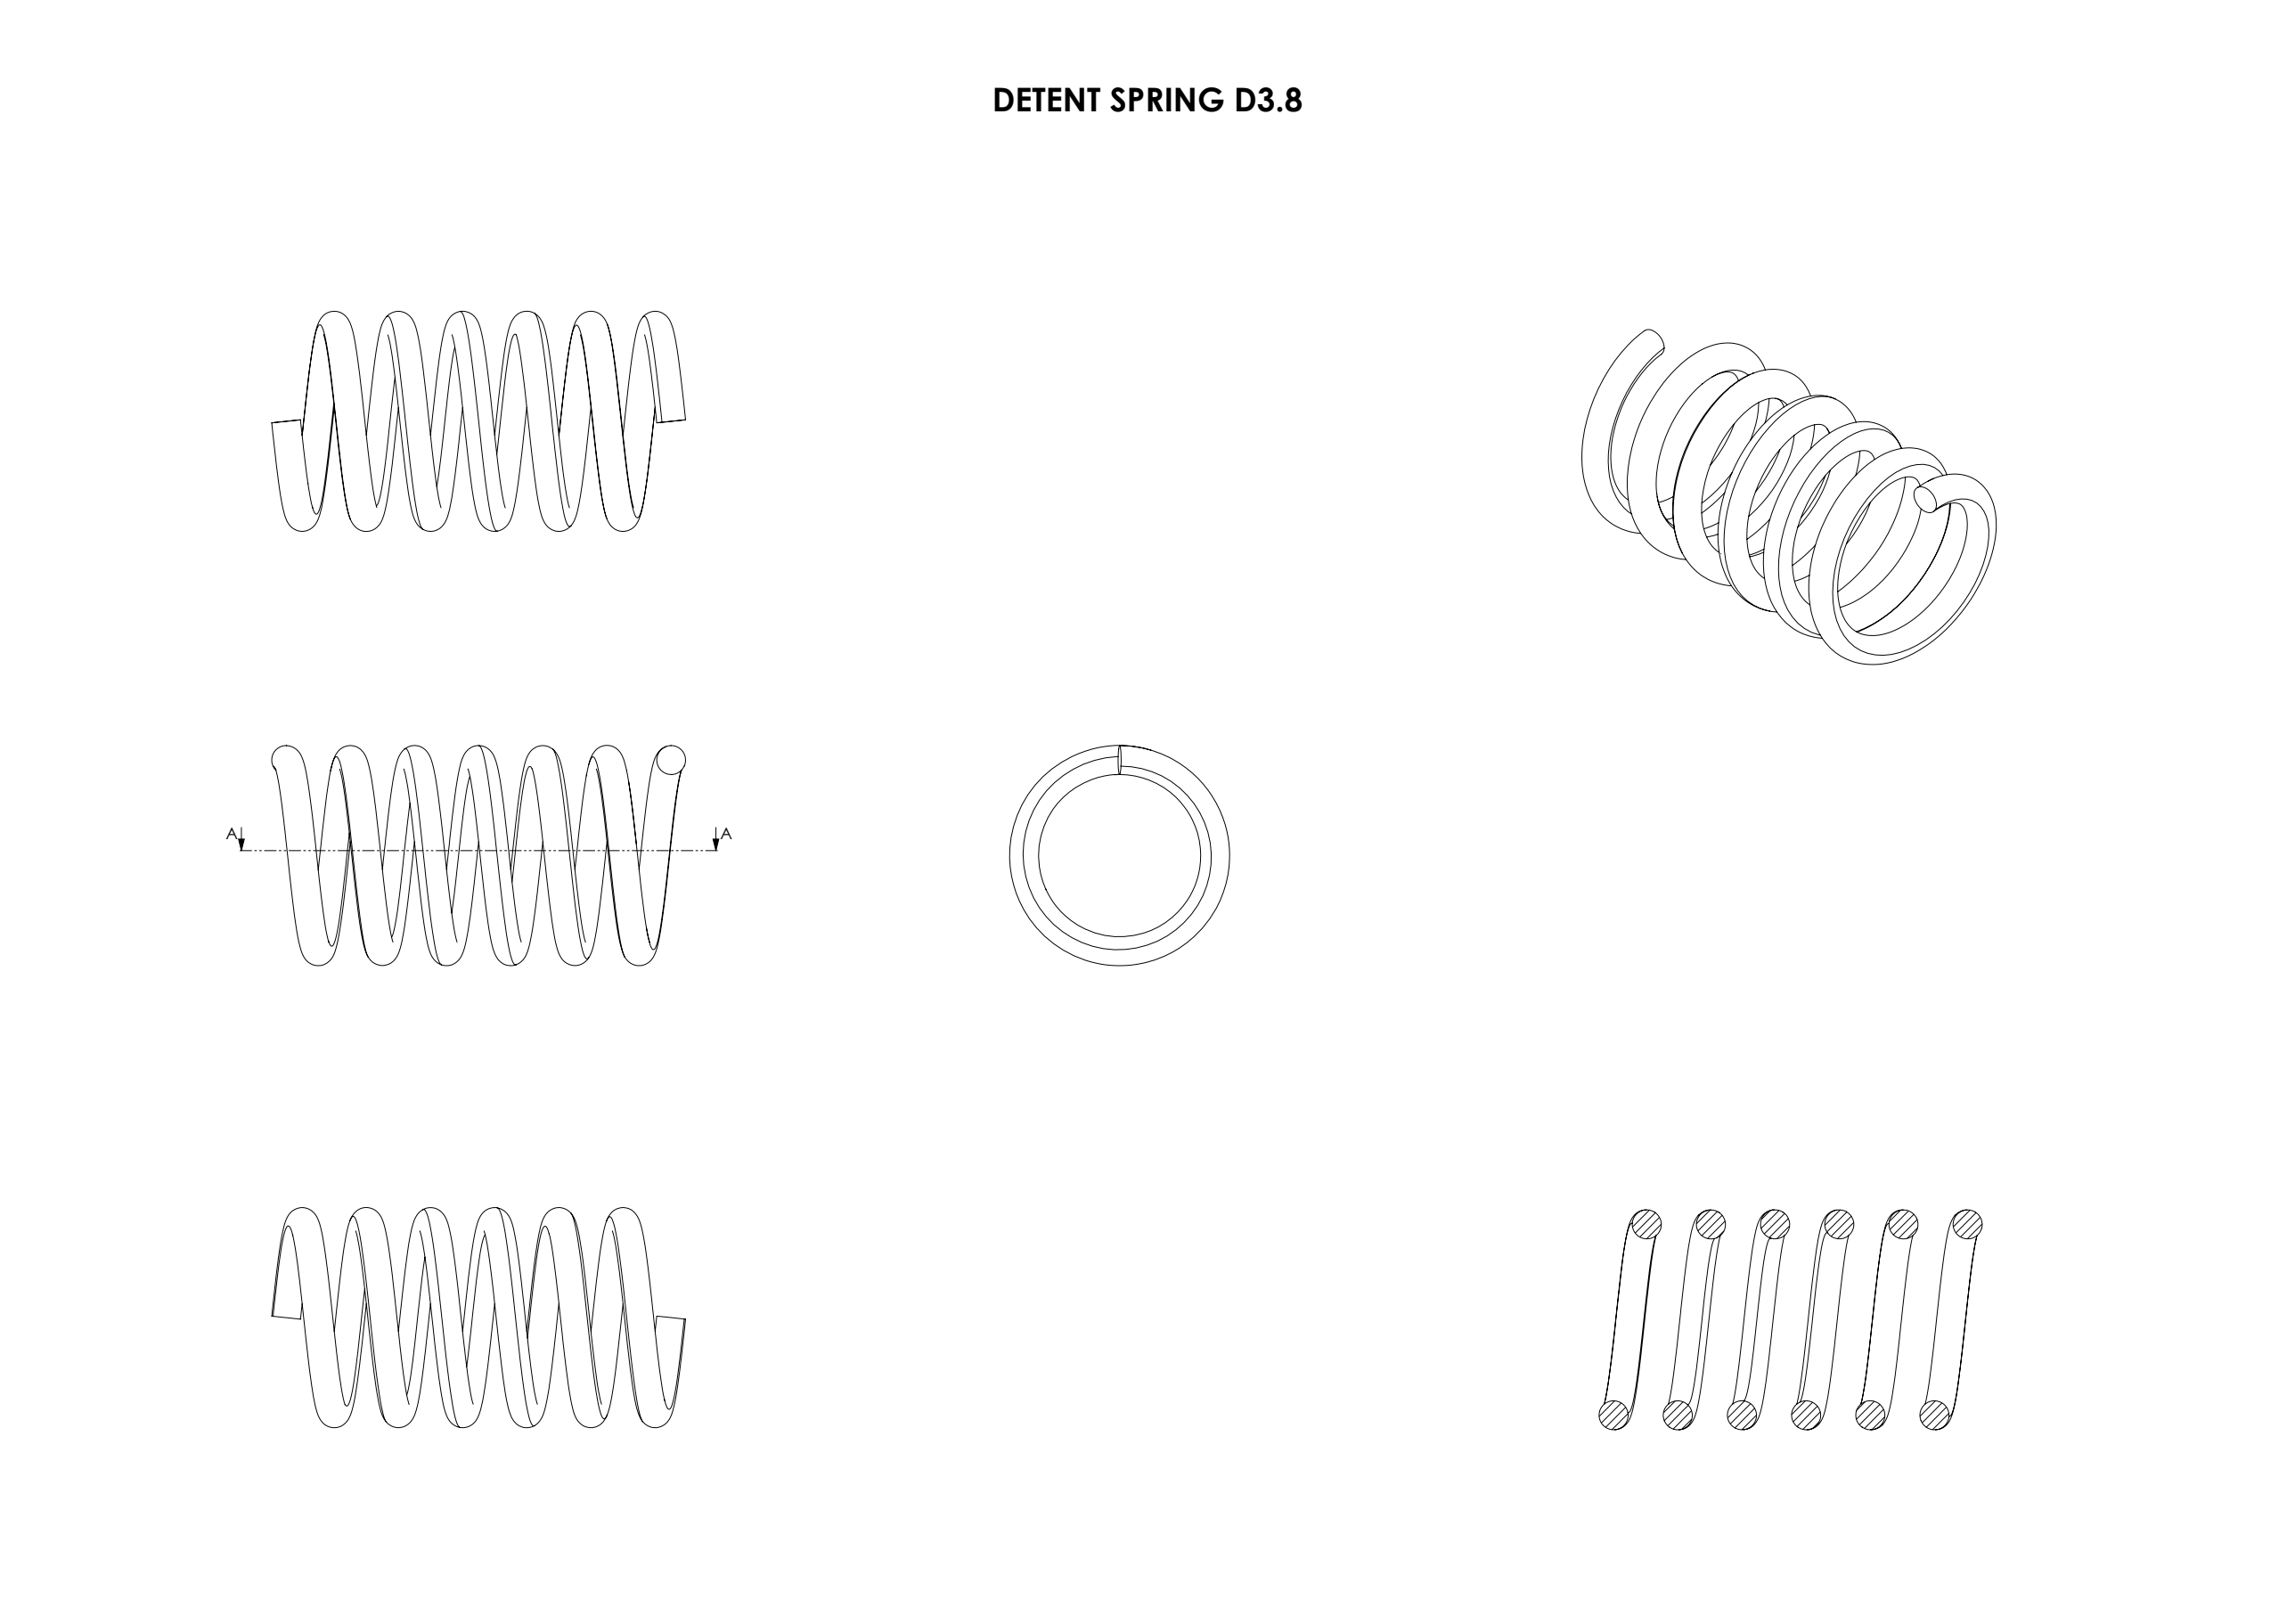
ISO-10303-21;
HEADER;
/* Generated by software containing ST-Developer
 * from STEP Tools, Inc. (www.steptools.com) 
 */

FILE_DESCRIPTION(
/* description */ (''),
/* implementation_level */ '2;1');

FILE_NAME(
/* name */ '10_Detent_Spring_D3.8.step',
/* time_stamp */ '2026-10-21T02:03:06-07:00',
/* author */ (''),
/* organization */ (''),
/* preprocessor_version */ 'ST-DEVELOPER v20.2',
/* originating_system */ 'Autodesk Translation Framework v15.15.0.0',
/* authorisation */ '');

FILE_SCHEMA (('AUTOMOTIVE_DESIGN { 1 0 10303 214 3 1 1 }'));
ENDSEC;

DATA;
#10=MECHANICAL_DESIGN_GEOMETRIC_PRESENTATION_REPRESENTATION('',(#124),#38528);
#86=B_SPLINE_SURFACE_WITH_KNOTS('',3,3,((#33827,#33828,#33829,#33830,#33831,
#33832,#33833,#33834,#33835,#33836,#33837,#33838,#33839,#33840,#33841,#33842,
#33843,#33844,#33845,#33846,#33847,#33848,#33849,#33850,#33851,#33852,#33853,
#33854,#33855,#33856,#33857,#33858,#33859,#33860,#33861,#33862,#33863,#33864,
#33865,#33866,#33867,#33868,#33869,#33870,#33871,#33872,#33873,#33874,#33875,
#33876,#33877,#33878,#33879,#33880,#33881,#33882,#33883,#33884,#33885,#33886,
#33887,#33888,#33889),(#33890,#33891,#33892,#33893,#33894,#33895,#33896,
#33897,#33898,#33899,#33900,#33901,#33902,#33903,#33904,#33905,#33906,#33907,
#33908,#33909,#33910,#33911,#33912,#33913,#33914,#33915,#33916,#33917,#33918,
#33919,#33920,#33921,#33922,#33923,#33924,#33925,#33926,#33927,#33928,#33929,
#33930,#33931,#33932,#33933,#33934,#33935,#33936,#33937,#33938,#33939,#33940,
#33941,#33942,#33943,#33944,#33945,#33946,#33947,#33948,#33949,#33950,#33951,
#33952),(#33953,#33954,#33955,#33956,#33957,#33958,#33959,#33960,#33961,
#33962,#33963,#33964,#33965,#33966,#33967,#33968,#33969,#33970,#33971,#33972,
#33973,#33974,#33975,#33976,#33977,#33978,#33979,#33980,#33981,#33982,#33983,
#33984,#33985,#33986,#33987,#33988,#33989,#33990,#33991,#33992,#33993,#33994,
#33995,#33996,#33997,#33998,#33999,#34000,#34001,#34002,#34003,#34004,#34005,
#34006,#34007,#34008,#34009,#34010,#34011,#34012,#34013,#34014,#34015),
(#34016,#34017,#34018,#34019,#34020,#34021,#34022,#34023,#34024,#34025,
#34026,#34027,#34028,#34029,#34030,#34031,#34032,#34033,#34034,#34035,#34036,
#34037,#34038,#34039,#34040,#34041,#34042,#34043,#34044,#34045,#34046,#34047,
#34048,#34049,#34050,#34051,#34052,#34053,#34054,#34055,#34056,#34057,#34058,
#34059,#34060,#34061,#34062,#34063,#34064,#34065,#34066,#34067,#34068,#34069,
#34070,#34071,#34072,#34073,#34074,#34075,#34076,#34077,#34078),(#34079,
#34080,#34081,#34082,#34083,#34084,#34085,#34086,#34087,#34088,#34089,#34090,
#34091,#34092,#34093,#34094,#34095,#34096,#34097,#34098,#34099,#34100,#34101,
#34102,#34103,#34104,#34105,#34106,#34107,#34108,#34109,#34110,#34111,#34112,
#34113,#34114,#34115,#34116,#34117,#34118,#34119,#34120,#34121,#34122,#34123,
#34124,#34125,#34126,#34127,#34128,#34129,#34130,#34131,#34132,#34133,#34134,
#34135,#34136,#34137,#34138,#34139,#34140,#34141),(#34142,#34143,#34144,
#34145,#34146,#34147,#34148,#34149,#34150,#34151,#34152,#34153,#34154,#34155,
#34156,#34157,#34158,#34159,#34160,#34161,#34162,#34163,#34164,#34165,#34166,
#34167,#34168,#34169,#34170,#34171,#34172,#34173,#34174,#34175,#34176,#34177,
#34178,#34179,#34180,#34181,#34182,#34183,#34184,#34185,#34186,#34187,#34188,
#34189,#34190,#34191,#34192,#34193,#34194,#34195,#34196,#34197,#34198,#34199,
#34200,#34201,#34202,#34203,#34204),(#34205,#34206,#34207,#34208,#34209,
#34210,#34211,#34212,#34213,#34214,#34215,#34216,#34217,#34218,#34219,#34220,
#34221,#34222,#34223,#34224,#34225,#34226,#34227,#34228,#34229,#34230,#34231,
#34232,#34233,#34234,#34235,#34236,#34237,#34238,#34239,#34240,#34241,#34242,
#34243,#34244,#34245,#34246,#34247,#34248,#34249,#34250,#34251,#34252,#34253,
#34254,#34255,#34256,#34257,#34258,#34259,#34260,#34261,#34262,#34263,#34264,
#34265,#34266,#34267),(#34268,#34269,#34270,#34271,#34272,#34273,#34274,
#34275,#34276,#34277,#34278,#34279,#34280,#34281,#34282,#34283,#34284,#34285,
#34286,#34287,#34288,#34289,#34290,#34291,#34292,#34293,#34294,#34295,#34296,
#34297,#34298,#34299,#34300,#34301,#34302,#34303,#34304,#34305,#34306,#34307,
#34308,#34309,#34310,#34311,#34312,#34313,#34314,#34315,#34316,#34317,#34318,
#34319,#34320,#34321,#34322,#34323,#34324,#34325,#34326,#34327,#34328,#34329,
#34330),(#34331,#34332,#34333,#34334,#34335,#34336,#34337,#34338,#34339,
#34340,#34341,#34342,#34343,#34344,#34345,#34346,#34347,#34348,#34349,#34350,
#34351,#34352,#34353,#34354,#34355,#34356,#34357,#34358,#34359,#34360,#34361,
#34362,#34363,#34364,#34365,#34366,#34367,#34368,#34369,#34370,#34371,#34372,
#34373,#34374,#34375,#34376,#34377,#34378,#34379,#34380,#34381,#34382,#34383,
#34384,#34385,#34386,#34387,#34388,#34389,#34390,#34391,#34392,#34393),
(#34394,#34395,#34396,#34397,#34398,#34399,#34400,#34401,#34402,#34403,
#34404,#34405,#34406,#34407,#34408,#34409,#34410,#34411,#34412,#34413,#34414,
#34415,#34416,#34417,#34418,#34419,#34420,#34421,#34422,#34423,#34424,#34425,
#34426,#34427,#34428,#34429,#34430,#34431,#34432,#34433,#34434,#34435,#34436,
#34437,#34438,#34439,#34440,#34441,#34442,#34443,#34444,#34445,#34446,#34447,
#34448,#34449,#34450,#34451,#34452,#34453,#34454,#34455,#34456),(#34457,
#34458,#34459,#34460,#34461,#34462,#34463,#34464,#34465,#34466,#34467,#34468,
#34469,#34470,#34471,#34472,#34473,#34474,#34475,#34476,#34477,#34478,#34479,
#34480,#34481,#34482,#34483,#34484,#34485,#34486,#34487,#34488,#34489,#34490,
#34491,#34492,#34493,#34494,#34495,#34496,#34497,#34498,#34499,#34500,#34501,
#34502,#34503,#34504,#34505,#34506,#34507,#34508,#34509,#34510,#34511,#34512,
#34513,#34514,#34515,#34516,#34517,#34518,#34519)),.UNSPECIFIED.,.T.,.F.,
 .F.,(4,1,1,1,1,1,1,1,4),(4,1,1,1,1,1,1,1,1,1,1,1,1,1,1,1,1,1,1,1,1,1,1,
1,1,1,1,1,1,1,1,1,1,1,1,1,1,1,1,1,1,1,1,1,1,1,1,1,1,1,1,1,1,1,1,1,1,1,1,
1,4),(-3.14159265358979,-2.46839422782055,-2.24399475256414,-1.34639685153848,
-0.448798950512828,0.448798950512828,1.34639685153848,2.24399475256414,
3.14159265358979),(0.,0.00892857142857143,0.0178571428571429,0.0357142857142857,
0.0535714285714286,0.0714285714285714,0.0892857142857143,0.107142857142857,
0.125,0.142857142857143,0.154761904761905,0.166666666666667,0.178571428571429,
0.19047619047619,0.202380952380952,0.214285714285714,0.238095238095238,
0.261904761904762,0.273809523809524,0.285714285714286,0.30952380952381,
0.333333333333333,0.357142857142857,0.369047619047619,0.380952380952381,
0.392857142857143,0.404761904761905,0.416666666666667,0.428571428571429,
0.446428571428571,0.464285714285714,0.482142857142857,0.5,0.517857142857143,
0.535714285714286,0.553571428571429,0.571428571428571,0.589285714285714,
0.607142857142857,0.625,0.642857142857143,0.660714285714286,0.678571428571428,
0.696428571428571,0.714285714285714,0.726190476190476,0.738095238095238,
0.761904761904762,0.785714285714286,0.809523809523809,0.833333333333333,
0.857142857142857,0.875,0.892857142857143,0.910714285714286,0.928571428571429,
0.946428571428571,0.964285714285714,0.982142857142857,0.991071428571429,
1.),.UNSPECIFIED.);
#100=SHAPE_REPRESENTATION_RELATIONSHIP('SRR','None',#38585,#112);
#112=ADVANCED_BREP_SHAPE_REPRESENTATION('',(#136),#38525);
#124=STYLED_ITEM('',(#38706),#136);
#136=MANIFOLD_SOLID_BREP('Body1',#17081);
#756=B_SPLINE_CURVE_WITH_KNOTS('',3,(#34523,#34524,#34525,#34526,#34527,
#34528,#34529,#34530,#34531,#34532,#34533,#34534,#34535,#34536,#34537,#34538,
#34539,#34540,#34541,#34542,#34543,#34544,#34545,#34546,#34547,#34548,#34549,
#34550,#34551,#34552,#34553,#34554,#34555,#34556,#34557,#34558,#34559,#34560,
#34561,#34562,#34563,#34564,#34565,#34566,#34567,#34568,#34569,#34570,#34571,
#34572,#34573,#34574,#34575,#34576,#34577,#34578,#34579,#34580,#34581,#34582,
#34583,#34584,#34585),.UNSPECIFIED.,.F.,.F.,(4,1,1,1,1,1,1,1,1,1,1,1,1,
1,1,1,1,1,1,1,1,1,1,1,1,1,1,1,1,1,1,1,1,1,1,1,1,1,1,1,1,1,1,1,1,1,1,1,1,
1,1,1,1,1,1,1,1,1,1,1,4),(0.,0.00892857142857143,0.0178571428571429,0.0357142857142857,
0.0535714285714286,0.0714285714285714,0.0892857142857143,0.107142857142857,
0.125,0.142857142857143,0.154761904761905,0.166666666666667,0.178571428571429,
0.19047619047619,0.202380952380952,0.214285714285714,0.238095238095238,
0.261904761904762,0.273809523809524,0.285714285714286,0.30952380952381,
0.333333333333333,0.357142857142857,0.369047619047619,0.380952380952381,
0.392857142857143,0.404761904761905,0.416666666666667,0.428571428571429,
0.446428571428571,0.464285714285714,0.482142857142857,0.5,0.517857142857143,
0.535714285714286,0.553571428571429,0.571428571428571,0.589285714285714,
0.607142857142857,0.625,0.642857142857143,0.660714285714286,0.678571428571428,
0.696428571428571,0.714285714285714,0.726190476190476,0.738095238095238,
0.761904761904762,0.785714285714286,0.809523809523809,0.833333333333333,
0.857142857142857,0.875,0.892857142857143,0.910714285714286,0.928571428571429,
0.946428571428571,0.964285714285714,0.982142857142857,0.991071428571429,
1.),.UNSPECIFIED.);
#2197=CIRCLE('',#18770,0.25);
#2198=CIRCLE('',#18771,0.25);
#3104=FACE_OUTER_BOUND('',#4130,.T.);
#3105=FACE_OUTER_BOUND('',#4131,.T.);
#3106=FACE_OUTER_BOUND('',#4132,.T.);
#4130=EDGE_LOOP('',(#14725,#14726,#14727,#14728));
#4131=EDGE_LOOP('',(#14729));
#4132=EDGE_LOOP('',(#14730));
#7587=VERTEX_POINT('',#34520);
#7588=VERTEX_POINT('',#34522);
#10014=EDGE_CURVE('',#7587,#7587,#2197,.T.);
#10015=EDGE_CURVE('',#7587,#7588,#756,.T.);
#10016=EDGE_CURVE('',#7588,#7588,#2198,.T.);
#14725=ORIENTED_EDGE('',*,*,#10014,.T.);
#14726=ORIENTED_EDGE('',*,*,#10015,.T.);
#14727=ORIENTED_EDGE('',*,*,#10016,.F.);
#14728=ORIENTED_EDGE('',*,*,#10015,.F.);
#14729=ORIENTED_EDGE('',*,*,#10016,.T.);
#14730=ORIENTED_EDGE('',*,*,#10014,.F.);
#15982=PLANE('',#18772);
#15983=PLANE('',#18773);
#16913=ADVANCED_FACE('',(#3104),#86,.T.);
#16914=ADVANCED_FACE('',(#3105),#15982,.T.);
#16915=ADVANCED_FACE('',(#3106),#15983,.F.);
#17081=CLOSED_SHELL('',(#16913,#16914,#16915));
#18769=AXIS2_PLACEMENT_3D('',#33826,#22893,#22894);
#18770=AXIS2_PLACEMENT_3D('',#34521,#22895,#22896);
#18771=AXIS2_PLACEMENT_3D('',#34586,#22897,#22898);
#18772=AXIS2_PLACEMENT_3D('',#34587,#22899,#22900);
#18773=AXIS2_PLACEMENT_3D('',#34588,#22901,#22902);
#22893=DIRECTION('axis',(0.,0.,1.));
#22894=DIRECTION('refdir',(1.,0.,0.));
#22895=DIRECTION('center_axis',(0.10451361405356,-0.00184126643092401,0.994521751504407));
#22896=DIRECTION('ref_axis',(-0.994367449791123,0.0175182479515601,0.104529832031847));
#22897=DIRECTION('center_axis',(0.104513613956506,0.00184126640140064,0.994521751514661));
#22898=DIRECTION('ref_axis',(0.631399161915391,-0.77273549595271,-0.0649226588123218));
#22899=DIRECTION('center_axis',(0.104513613956506,0.00184126640140064,0.994521751514661));
#22900=DIRECTION('ref_axis',(0.631399161915391,-0.77273549595271,-0.0649226588123217));
#22901=DIRECTION('center_axis',(0.10451361405356,-0.00184126643092401,0.994521751504407));
#22902=DIRECTION('ref_axis',(-0.994367449791123,0.0175182479515601,0.104529832031847));
#33826=CARTESIAN_POINT('',(0.,0.,0.));
#33827=CARTESIAN_POINT('Ctrl Pts',(0.508591862447781,1.64562043801211,-0.0261324580079617));
#33828=CARTESIAN_POINT('Ctrl Pts',(0.528271024599208,1.6452737407805,0.161128837931408));
#33829=CARTESIAN_POINT('Ctrl Pts',(0.567647573513685,1.58281094560678,0.524492831752905));
#33830=CARTESIAN_POINT('Ctrl Pts',(0.645996560435206,1.22365592193525,1.1787804941138));
#33831=CARTESIAN_POINT('Ctrl Pts',(0.743073641882897,0.410281924307437,
1.68766009875447));
#33832=CARTESIAN_POINT('Ctrl Pts',(0.858352417401347,-0.724396860085975,
1.55831173688398));
#33833=CARTESIAN_POINT('Ctrl Pts',(0.972375295448021,-1.52098532662473,
0.758217612597792));
#33834=CARTESIAN_POINT('Ctrl Pts',(1.08519171777668,-1.64409811634449,-0.352032188510366));
#33835=CARTESIAN_POINT('Ctrl Pts',(1.19681996654867,-1.05450947578872,-1.28675893283186));
#33836=CARTESIAN_POINT('Ctrl Pts',(1.30730161177351,-0.0208333311052113,
-1.64663068201152));
#33837=CARTESIAN_POINT('Ctrl Pts',(1.40452364629174,0.886236470079679,-1.32621345051066));
#33838=CARTESIAN_POINT('Ctrl Pts',(1.48890750188156,1.38959463750653,-0.691912415510853));
#33839=CARTESIAN_POINT('Ctrl Pts',(1.56078188611823,1.54308896603543,-0.0198177610475133));
#33840=CARTESIAN_POINT('Ctrl Pts',(1.63221817171176,1.38983552550406,0.647948130516392));
#33841=CARTESIAN_POINT('Ctrl Pts',(1.70323404319384,0.964738946565908,1.1812205675546));
#33842=CARTESIAN_POINT('Ctrl Pts',(1.77384798276294,0.354991450441324,1.47260961294232));
#33843=CARTESIAN_POINT('Ctrl Pts',(1.86748993119896,-0.546099502039117,
1.47825694934893));
#33844=CARTESIAN_POINT('Ctrl Pts',(1.98363667823136,-1.48203264186415,0.7293081873873));
#33845=CARTESIAN_POINT('Ctrl Pts',(2.09871900316068,-1.48120258062414,-0.462340692211473));
#33846=CARTESIAN_POINT('Ctrl Pts',(2.19023826573612,-0.927379733426102,
-1.14481302651884));
#33847=CARTESIAN_POINT('Ctrl Pts',(2.2814255547235,-0.141378759287938,-1.52891931607764));
#33848=CARTESIAN_POINT('Ctrl Pts',(2.39484749559815,1.00382275253285,-1.27061478852019));
#33849=CARTESIAN_POINT('Ctrl Pts',(2.53025681997088,1.60865186335246,-0.00254459019504153));
#33850=CARTESIAN_POINT('Ctrl Pts',(2.64269039045238,1.10418776314993,1.04117197496908));
#33851=CARTESIAN_POINT('Ctrl Pts',(2.73249952801582,0.322974585676589,1.41105820876749));
#33852=CARTESIAN_POINT('Ctrl Pts',(2.7998141074244,-0.32110895921182,1.41232437949226));
#33853=CARTESIAN_POINT('Ctrl Pts',(2.86711382621074,-0.903428721470414,
1.13164638734841));
#33854=CARTESIAN_POINT('Ctrl Pts',(2.93442516377676,-1.30601623783849,0.626923391067463));
#33855=CARTESIAN_POINT('Ctrl Pts',(3.00177556402078,-1.44931171614156,-0.00280700337714968));
#33856=CARTESIAN_POINT('Ctrl Pts',(3.08042754178598,-1.28252605621248,-0.73905091180395));
#33857=CARTESIAN_POINT('Ctrl Pts',(3.17046965462109,-0.654511755766728,
-1.3704712298758));
#33858=CARTESIAN_POINT('Ctrl Pts',(3.27206448378161,0.346719679199525,-1.483704431146));
#33859=CARTESIAN_POINT('Ctrl Pts',(3.3740442463093,1.20102786916375,-0.946430056825302));
#33860=CARTESIAN_POINT('Ctrl Pts',(3.47649477143674,1.53732148053407,0.0107120740773195));
#33861=CARTESIAN_POINT('Ctrl Pts',(3.57949954098879,1.20134163447082,0.973667458417707));
#33862=CARTESIAN_POINT('Ctrl Pts',(3.68313928551533,0.333095090941954,1.52059902024328));
#33863=CARTESIAN_POINT('Ctrl Pts',(3.78749120379714,-0.693842597912142,
1.40614340263662));
#33864=CARTESIAN_POINT('Ctrl Pts',(3.89262893585172,-1.43094857905026,0.670971912346831));
#33865=CARTESIAN_POINT('Ctrl Pts',(3.99862203011025,-1.5499543985351,-0.371794281933162));
#33866=CARTESIAN_POINT('Ctrl Pts',(4.10553567293418,-0.988090997030439,
-1.26903707993744));
#33867=CARTESIAN_POINT('Ctrl Pts',(4.21343045112327,0.0197202801860453,
-1.62347464599002));
#33868=CARTESIAN_POINT('Ctrl Pts',(4.32236196180067,1.03832038776908,-1.26894288895586));
#33869=CARTESIAN_POINT('Ctrl Pts',(4.43238051112357,1.61925828890368,-0.34739423883176));
#33870=CARTESIAN_POINT('Ctrl Pts',(4.54353062752128,1.4989897755625,0.74620181404568));
#33871=CARTESIAN_POINT('Ctrl Pts',(4.65585125526312,0.71351870218781,1.53444845290457));
#33872=CARTESIAN_POINT('Ctrl Pts',(4.75676135685292,-0.279697500338493,
1.64729603227415));
#33873=CARTESIAN_POINT('Ctrl Pts',(4.84585493867587,-1.04780204615629,1.27474307821934));
#33874=CARTESIAN_POINT('Ctrl Pts',(4.94841313843452,-1.66845031883017,0.508931034591464));
#33875=CARTESIAN_POINT('Ctrl Pts',(5.07800659502253,-1.67475443904525,-0.829467776745351));
#33876=CARTESIAN_POINT('Ctrl Pts',(5.23577771702336,-0.399579932550961,
-1.85373353020478));
#33877=CARTESIAN_POINT('Ctrl Pts',(5.39581269472486,1.21472097060722,-1.48922395511139));
#33878=CARTESIAN_POINT('Ctrl Pts',(5.55809610080897,1.95203227446324,0.0217272724024816));
#33879=CARTESIAN_POINT('Ctrl Pts',(5.70888367040444,1.27533356599845,1.42745494534175));
#33880=CARTESIAN_POINT('Ctrl Pts',(5.84753617842438,-0.0234051752573978,
1.87960329280061));
#33881=CARTESIAN_POINT('Ctrl Pts',(5.9735033792588,-1.2000636353636,1.47084402209574));
#33882=CARTESIAN_POINT('Ctrl Pts',(6.10061934653175,-1.87205652425054,0.4054527917675));
#33883=CARTESIAN_POINT('Ctrl Pts',(6.22882892874595,-1.73128184695155,-0.856020464879398));
#33884=CARTESIAN_POINT('Ctrl Pts',(6.35811249074499,-0.82796691613823,-1.76256406416465));
#33885=CARTESIAN_POINT('Ctrl Pts',(6.48835538046169,0.454518312141212,-1.90827828922266));
#33886=CARTESIAN_POINT('Ctrl Pts',(6.59776527270895,1.37009311469038,-1.33377327146165));
#33887=CARTESIAN_POINT('Ctrl Pts',(6.68557306476182,1.77276616876359,-0.600525447669764));
#33888=CARTESIAN_POINT('Ctrl Pts',(6.72979494253028,1.84279755540219,-0.192431284750887));
#33889=CARTESIAN_POINT('Ctrl Pts',(6.75172308477496,1.84318387398818,0.016230664703078));
#33890=CARTESIAN_POINT('Ctrl Pts',(0.509580047382347,1.70171160283773,-0.0261324580079617));
#33891=CARTESIAN_POINT('Ctrl Pts',(0.529895087764518,1.70135370303456,0.167179673868041));
#33892=CARTESIAN_POINT('Ctrl Pts',(0.570639757970856,1.63675411705557,0.543184963069467));
#33893=CARTESIAN_POINT('Ctrl Pts',(0.6516200225759,1.26545922887677,1.21943960034875));
#33894=CARTESIAN_POINT('Ctrl Pts',(0.752012920500956,0.424415974257467,
1.74584191963726));
#33895=CARTESIAN_POINT('Ctrl Pts',(0.871203035093005,-0.748901033499195,
1.61196056324099));
#33896=CARTESIAN_POINT('Ctrl Pts',(0.989080507646655,-1.57236986743728,
0.784770914561726));
#33897=CARTESIAN_POINT('Ctrl Pts',(1.10566189091232,-1.69947969245876,-0.362632153218937));
#33898=CARTESIAN_POINT('Ctrl Pts',(1.22095215672461,-1.09039676853272,-1.32796705536343));
#33899=CARTESIAN_POINT('Ctrl Pts',(1.33497129130756,-0.0235221960857565,
-1.69919666569563));
#33900=CARTESIAN_POINT('Ctrl Pts',(1.43521215485341,0.911646464020701,-1.36863402635081));
#33901=CARTESIAN_POINT('Ctrl Pts',(1.52213389548391,1.43007830855258,-0.715200055347309));
#33902=CARTESIAN_POINT('Ctrl Pts',(1.59610957693942,1.58797356382673,-0.0234496931959115));
#33903=CARTESIAN_POINT('Ctrl Pts',(1.6695643364048,1.43030938586697,0.663167430554008));
#33904=CARTESIAN_POINT('Ctrl Pts',(1.74251566986873,0.993555991276766,1.21088878338602));
#33905=CARTESIAN_POINT('Ctrl Pts',(1.81497296241828,0.367875249236745,1.50980906152487));
#33906=CARTESIAN_POINT('Ctrl Pts',(1.91095320023966,-0.555718724718245,
1.51541429690618));
#33907=CARTESIAN_POINT('Ctrl Pts',(2.02977137858219,-1.51271899954516,0.748724773148181));
#33908=CARTESIAN_POINT('Ctrl Pts',(2.14718490518103,-1.51104304623224,-0.466989387116428));
#33909=CARTESIAN_POINT('Ctrl Pts',(2.24034153374774,-0.94726476473438,-1.16142922577992));
#33910=CARTESIAN_POINT('Ctrl Pts',(2.33300573809692,-0.148443790584567,
-1.5516251873687));
#33911=CARTESIAN_POINT('Ctrl Pts',(2.44801880375704,1.01237692380644,-1.28879026893535));
#33912=CARTESIAN_POINT('Ctrl Pts',(2.58481878669611,1.62223628112757,-0.00735339085508992));
#33913=CARTESIAN_POINT('Ctrl Pts',(2.69799779409897,1.11364043446412,1.04273258659252));
#33914=CARTESIAN_POINT('Ctrl Pts',(2.78815431916423,0.329470398073438,1.41374437778883));
#33915=CARTESIAN_POINT('Ctrl Pts',(2.85560391946039,-0.315812807091245,
1.41487913006738));
#33916=CARTESIAN_POINT('Ctrl Pts',(2.92290913292631,-0.898041393277587,
1.13407835691753));
#33917=CARTESIAN_POINT('Ctrl Pts',(2.99010748782479,-1.29975039474633,0.630211173964469));
#33918=CARTESIAN_POINT('Ctrl Pts',(3.05720153737446,-1.44237298019696,0.00291322106573988));
#33919=CARTESIAN_POINT('Ctrl Pts',(3.13540758721451,-1.27637311566389,-0.729048078712233));
#33920=CARTESIAN_POINT('Ctrl Pts',(3.22474166887994,-0.653103075230279,
-1.35515277979788));
#33921=CARTESIAN_POINT('Ctrl Pts',(3.32529053184942,0.337558356289205,-1.46669075353571));
#33922=CARTESIAN_POINT('Ctrl Pts',(3.42590699610091,1.18013302272422,-0.936320642038885));
#33923=CARTESIAN_POINT('Ctrl Pts',(3.52675591022479,1.5106801904221,0.00578391821411416));
#33924=CARTESIAN_POINT('Ctrl Pts',(3.62789543596507,1.1804735150479,0.950962905372855));
#33925=CARTESIAN_POINT('Ctrl Pts',(3.72942248398239,0.329909659532609,1.48630965540244));
#33926=CARTESIAN_POINT('Ctrl Pts',(3.83142370458731,-0.673643861606902,
1.37409910302327));
#33927=CARTESIAN_POINT('Ctrl Pts',(3.93398592718664,-1.39230980841848,0.656853426449074));
#33928=CARTESIAN_POINT('Ctrl Pts',(4.03719172387346,-1.50786192508977,-0.358317467730407));
#33929=CARTESIAN_POINT('Ctrl Pts',(4.14112075232382,-0.961565622810986,
-1.23019350319165));
#33930=CARTESIAN_POINT('Ctrl Pts',(4.24584932913355,0.0165600109717206,
-1.57393537894064));
#33931=CARTESIAN_POINT('Ctrl Pts',(4.35144915285955,1.00374162047219,-1.23012207438448));
#33932=CARTESIAN_POINT('Ctrl Pts',(4.4579909264812,1.56609007503267,-0.337790096423364));
#33933=CARTESIAN_POINT('Ctrl Pts',(4.56551149543496,1.44958631126263,0.719976289482437));
#33934=CARTESIAN_POINT('Ctrl Pts',(4.67411908241366,0.69021449004645,1.48194813108531));
#33935=CARTESIAN_POINT('Ctrl Pts',(4.77164000284681,-0.26949798097472,1.59091301338937));
#33936=CARTESIAN_POINT('Ctrl Pts',(4.85771048721972,-1.01144589727057,1.23104757178239));
#33937=CARTESIAN_POINT('Ctrl Pts',(4.9567809680996,-1.61090774880558,0.491362209635852));
#33938=CARTESIAN_POINT('Ctrl Pts',(5.08196285876115,-1.61704639101494,-0.801332081949465));
#33939=CARTESIAN_POINT('Ctrl Pts',(5.23440617825647,-0.385186946102618,
-1.79103900031212));
#33940=CARTESIAN_POINT('Ctrl Pts',(5.38912164940439,1.17539727930777,-1.43897710296556));
#33941=CARTESIAN_POINT('Ctrl Pts',(5.54614784502495,1.88913047177666,0.0227340869851706));
#33942=CARTESIAN_POINT('Ctrl Pts',(5.69223084261495,1.23407058093322,1.38466393862149));
#33943=CARTESIAN_POINT('Ctrl Pts',(5.82670511437593,-0.0254194746735188,
1.82344694793182));
#33944=CARTESIAN_POINT('Ctrl Pts',(5.94902331756535,-1.1680230768833,1.42680551782825));
#33945=CARTESIAN_POINT('Ctrl Pts',(6.07261244268437,-1.82162602449473,0.391140168157498));
#33946=CARTESIAN_POINT('Ctrl Pts',(6.19744218367146,-1.68489344120707,-0.837072796063665));
#33947=CARTESIAN_POINT('Ctrl Pts',(6.32349906024936,-0.804352968952716,
-1.72132362315681));
#33948=CARTESIAN_POINT('Ctrl Pts',(6.45070645344015,0.448136825520351,-1.86394181546585));
#33949=CARTESIAN_POINT('Ctrl Pts',(6.55771675748864,1.343944695716,-1.30238352555007));
#33950=CARTESIAN_POINT('Ctrl Pts',(6.64375918572647,1.73853556054087,-0.583881007842722));
#33951=CARTESIAN_POINT('Ctrl Pts',(6.68709903227955,1.80719676573851,-0.1839314494448));
#33952=CARTESIAN_POINT('Ctrl Pts',(6.70861691504104,1.80757585658667,0.0208265877402715));
#33953=CARTESIAN_POINT('Ctrl Pts',(0.48473626150267,1.77644942930338,-0.0233832711793042));
#33954=CARTESIAN_POINT('Ctrl Pts',(0.505893844496287,1.7760766860232,0.177946255954152));
#33955=CARTESIAN_POINT('Ctrl Pts',(0.548463328130588,1.70860250247314,0.570776926736889));
#33956=CARTESIAN_POINT('Ctrl Pts',(0.632982327171215,1.32101158554047,1.27654377010548));
#33957=CARTESIAN_POINT('Ctrl Pts',(0.737996501360194,0.441739014073499,
1.82746202052102));
#33958=CARTESIAN_POINT('Ctrl Pts',(0.862723494828206,-0.786157377851955,
1.68745064871946));
#33959=CARTESIAN_POINT('Ctrl Pts',(0.986209664727694,-1.64882413818832,
0.821304842815863));
#33960=CARTESIAN_POINT('Ctrl Pts',(1.10839876372818,-1.78218917322355,-0.381247653647888));
#33961=CARTESIAN_POINT('Ctrl Pts',(1.22928857352045,-1.14366016506855,-1.39342331335522));
#33962=CARTESIAN_POINT('Ctrl Pts',(1.34886146417612,-0.0248717421322719,
-1.78277108349345));
#33963=CARTESIAN_POINT('Ctrl Pts',(1.45397742207399,0.955759686067741,-1.4361457574584));
#33964=CARTESIAN_POINT('Ctrl Pts',(1.54509991200394,1.49922256563711,-0.751131218932962));
#33965=CARTESIAN_POINT('Ctrl Pts',(1.62262212832639,1.66468393757921,-0.0261951730747789));
#33966=CARTESIAN_POINT('Ctrl Pts',(1.69956649110401,1.49950125883268,0.693032382528641));
#33967=CARTESIAN_POINT('Ctrl Pts',(1.77593637879585,1.04223323460681,1.26643212720561));
#33968=CARTESIAN_POINT('Ctrl Pts',(1.85174001831755,0.387640963552032,1.57911778202419));
#33969=CARTESIAN_POINT('Ctrl Pts',(1.95206329984898,-0.577882239813857,
1.58491583806782));
#33970=CARTESIAN_POINT('Ctrl Pts',(2.07609288529357,-1.57652280363707,0.784118879423183));
#33971=CARTESIAN_POINT('Ctrl Pts',(2.19835334034983,-1.57411269447054,-0.481987546861393));
#33972=CARTESIAN_POINT('Ctrl Pts',(2.29515759309052,-0.988081044302533,
-1.20354579776995));
#33973=CARTESIAN_POINT('Ctrl Pts',(2.39131513088785,-0.158981373237876,
-1.6083713901134));
#33974=CARTESIAN_POINT('Ctrl Pts',(2.5103164166735,1.04239264391016,-1.33544690779909));
#33975=CARTESIAN_POINT('Ctrl Pts',(2.65138524018481,1.67017090611041,-0.0133144094548457));
#33976=CARTESIAN_POINT('Ctrl Pts',(2.76761689590905,1.14685339948012,1.06483740920086));
#33977=CARTESIAN_POINT('Ctrl Pts',(2.85989151047589,0.344054458745719,1.44437130805655));
#33978=CARTESIAN_POINT('Ctrl Pts',(2.92876498103789,-0.315007838050914,
1.44542580052931));
#33979=CARTESIAN_POINT('Ctrl Pts',(2.99733123089316,-0.908178327495592,
1.1591356196893));
#33980=CARTESIAN_POINT('Ctrl Pts',(3.065609203041,-1.31633070800262,0.646932225733396));
#33981=CARTESIAN_POINT('Ctrl Pts',(3.13363492285534,-1.46075866519691,0.0108009638378416));
#33982=CARTESIAN_POINT('Ctrl Pts',(3.2127246664228,-1.29265108627793,-0.729519994292884));
#33983=CARTESIAN_POINT('Ctrl Pts',(3.30276107775906,-0.663900215810431,
-1.36029592969158));
#33984=CARTESIAN_POINT('Ctrl Pts',(3.40366000172583,0.330744582477941,-1.47158912535297));
#33985=CARTESIAN_POINT('Ctrl Pts',(3.50428991474366,1.17315483841855,-0.940484753739533));
#33986=CARTESIAN_POINT('Ctrl Pts',(3.60471206445919,1.50180382114359,-0.00182149644391336));
#33987=CARTESIAN_POINT('Ctrl Pts',(3.70503499179928,1.1735346580546,0.935792533952136));
#33988=CARTESIAN_POINT('Ctrl Pts',(3.8053502869075,0.332515303599265,1.46435790052267));
#33989=CARTESIAN_POINT('Ctrl Pts',(3.90575276069741,-0.655532733693565,
1.35324201618498));
#33990=CARTESIAN_POINT('Ctrl Pts',(4.0063357525127,-1.36010254886635,0.649193189923515));
#33991=CARTESIAN_POINT('Ctrl Pts',(4.10719217500436,-1.47247077545791,-0.343223377561497));
#33992=CARTESIAN_POINT('Ctrl Pts',(4.20841335510511,-0.939776138769746,
-1.1923257631531));
#33993=CARTESIAN_POINT('Ctrl Pts',(4.31008881701827,0.0102721264493911,
-1.52564233507173));
#33994=CARTESIAN_POINT('Ctrl Pts',(4.41230607006117,0.965941125693951,-1.19227951792117));
#33995=CARTESIAN_POINT('Ctrl Pts',(4.51514840136008,1.50849130946414,-0.330439751053724));
#33996=CARTESIAN_POINT('Ctrl Pts',(4.61870840436037,1.39590489437915,0.688474310705198));
#33997=CARTESIAN_POINT('Ctrl Pts',(4.7230411604876,0.665865263436382,1.42037460677782));
#33998=CARTESIAN_POINT('Ctrl Pts',(4.81654767173681,-0.254564879881144,
1.52461360384059));
#33999=CARTESIAN_POINT('Ctrl Pts',(4.89897224099944,-0.965161399415059,
1.17984498732178));
#34000=CARTESIAN_POINT('Ctrl Pts',(4.99374606403791,-1.53863694276043,0.472007785395054));
#34001=CARTESIAN_POINT('Ctrl Pts',(5.11333980190992,-1.54407067005438,-0.763171998627613));
#34002=CARTESIAN_POINT('Ctrl Pts',(5.25878882582696,-0.368307274360266,
-1.70728369755521));
#34003=CARTESIAN_POINT('Ctrl Pts',(5.40629446830278,1.11962985036899,-1.3713425153718));
#34004=CARTESIAN_POINT('Ctrl Pts',(5.55595232991783,1.79986048336761,0.021931639638948));
#34005=CARTESIAN_POINT('Ctrl Pts',(5.69517763482324,1.17545690153292,1.32014816214982));
#34006=CARTESIAN_POINT('Ctrl Pts',(5.82342289422373,-0.0257032202752489,
1.73872373843064));
#34007=CARTESIAN_POINT('Ctrl Pts',(5.94014607560228,-1.11615143607484,1.36030281643229));
#34008=CARTESIAN_POINT('Ctrl Pts',(6.05818632607282,-1.74056421947656,0.371182103626331));
#34009=CARTESIAN_POINT('Ctrl Pts',(6.17754324250935,-1.61002629882336,-0.80318878992352));
#34010=CARTESIAN_POINT('Ctrl Pts',(6.29822057589678,-0.767189384090067,
-1.64997568303796));
#34011=CARTESIAN_POINT('Ctrl Pts',(6.42019478496613,0.433634258784792,-1.78689227136282));
#34012=CARTESIAN_POINT('Ctrl Pts',(6.52293527463248,1.29405210388765,-1.24809073369933));
#34013=CARTESIAN_POINT('Ctrl Pts',(6.60571721409053,1.67365883220886,-0.556808735892081));
#34014=CARTESIAN_POINT('Ctrl Pts',(6.64739595189646,1.73973417470393,-0.172198300266751));
#34015=CARTESIAN_POINT('Ctrl Pts',(6.66814094153175,1.74009964912365,0.0252051062964792));
#34016=CARTESIAN_POINT('Ctrl Pts',(0.381117442983887,1.88549148283562,-0.0122921586285728));
#34017=CARTESIAN_POINT('Ctrl Pts',(0.403532825828836,1.88509658029261,0.20100623325534));
#34018=CARTESIAN_POINT('Ctrl Pts',(0.448799900969048,1.81344132117068,0.618761006536107));
#34019=CARTESIAN_POINT('Ctrl Pts',(0.538679332142541,1.40127335864296,1.36930440711935));
#34020=CARTESIAN_POINT('Ctrl Pts',(0.650838448754394,0.46290690991,1.95859094615097));
#34021=CARTESIAN_POINT('Ctrl Pts',(0.784506730841078,-0.853342453722629,
1.80916959778172));
#34022=CARTESIAN_POINT('Ctrl Pts',(0.917364661912327,-1.78200024295873,
0.877975354207177));
#34023=CARTESIAN_POINT('Ctrl Pts',(1.04926270425752,-1.92666667943644,-0.420181769112088));
#34024=CARTESIAN_POINT('Ctrl Pts',(1.18017007182846,-1.23574698396432,-1.51656075807354));
#34025=CARTESIAN_POINT('Ctrl Pts',(1.31000892844173,-0.0210398826096366,
-1.93988507897714));
#34026=CARTESIAN_POINT('Ctrl Pts',(1.42442730051466,1.0465288908201,-1.56293923922871));
#34027=CARTESIAN_POINT('Ctrl Pts',(1.52378385033388,1.63922012112484,-0.816087647064672));
#34028=CARTESIAN_POINT('Ctrl Pts',(1.60841315506779,1.81993148953039,-0.0247216582983172));
#34029=CARTESIAN_POINT('Ctrl Pts',(1.69249524019256,1.63950112746236,0.761246734592579));
#34030=CARTESIAN_POINT('Ctrl Pts',(1.77602032928508,1.1394414206172,1.38839301192058));
#34031=CARTESIAN_POINT('Ctrl Pts',(1.85897694842633,0.423103070241056,1.73061206360768));
#34032=CARTESIAN_POINT('Ctrl Pts',(1.96881924664199,-0.634001252397349,
1.73700910342183));
#34033=CARTESIAN_POINT('Ctrl Pts',(2.10466048128153,-1.72773172837744,0.859962453630954));
#34034=CARTESIAN_POINT('Ctrl Pts',(2.23852274988566,-1.72484281980162,-0.526238676081834));
#34035=CARTESIAN_POINT('Ctrl Pts',(2.34441167003019,-1.08376675443436,-1.31536550154628));
#34036=CARTESIAN_POINT('Ctrl Pts',(2.44949842855696,-0.177626983089426,
-1.75770921156832));
#34037=CARTESIAN_POINT('Ctrl Pts',(2.57936886683961,1.13316325023126,-1.45907163886627));
#34038=CARTESIAN_POINT('Ctrl Pts',(2.73282739757898,1.81479123414694,-0.0203495029752695));
#34039=CARTESIAN_POINT('Ctrl Pts',(2.85876666181656,1.24669618273856,1.14720091126386));
#34040=CARTESIAN_POINT('Ctrl Pts',(2.95838625405263,0.379992571081585,1.55652976858396));
#34041=CARTESIAN_POINT('Ctrl Pts',(3.03254530339479,-0.329577958511324,
1.55746711909117));
#34042=CARTESIAN_POINT('Ctrl Pts',(3.10615895005409,-0.96625312134884,1.24989533056844));
#34043=CARTESIAN_POINT('Ctrl Pts',(3.17924306329434,-1.40286089813684,0.701552239452624));
#34044=CARTESIAN_POINT('Ctrl Pts',(3.25180396600809,-1.55666651553022,0.0230087966776739));
#34045=CARTESIAN_POINT('Ctrl Pts',(3.33587136562189,-1.37764426396791,-0.763794702731238));
#34046=CARTESIAN_POINT('Ctrl Pts',(3.43113975717292,-0.711774228624347,
-1.4305765381498));
#34047=CARTESIAN_POINT('Ctrl Pts',(3.5372886042444,0.334525637087803,-1.54647218216131));
#34048=CARTESIAN_POINT('Ctrl Pts',(3.64245111618431,1.21419218905581,-0.990566084988547));
#34049=CARTESIAN_POINT('Ctrl Pts',(3.74671900888706,1.55424048357597,-0.0157101568300266));
#34050=CARTESIAN_POINT('Ctrl Pts',(3.85015607940294,1.21467035959478,0.950447047776102));
#34051=CARTESIAN_POINT('Ctrl Pts',(3.9528428913112,0.353239193399766,1.49035956049266));
#34052=CARTESIAN_POINT('Ctrl Pts',(4.05486113278981,-0.650409675441866,
1.37619957489024));
#34053=CARTESIAN_POINT('Ctrl Pts',(4.15629674336446,-1.35992778763908,0.665383226257766));
#34054=CARTESIAN_POINT('Ctrl Pts',(4.25723817727952,-1.47109033257279,-0.327860133764075));
#34055=CARTESIAN_POINT('Ctrl Pts',(4.35777648370015,-0.940986099129111,
-1.17042124327949));
#34056=CARTESIAN_POINT('Ctrl Pts',(4.45800500695589,-0.00418280368968732,
-1.49774982508127));
#34057=CARTESIAN_POINT('Ctrl Pts',(4.5580185838917,0.930328530149581,-1.17045669235878));
#34058=CARTESIAN_POINT('Ctrl Pts',(4.65791431280149,1.45624348325976,-0.332815962728341));
#34059=CARTESIAN_POINT('Ctrl Pts',(4.75778043706964,1.34650681780447,0.649575118733562));
#34060=CARTESIAN_POINT('Ctrl Pts',(4.85772972138868,0.646482048134813,1.3498091217411));
#34061=CARTESIAN_POINT('Ctrl Pts',(4.94672281509739,-0.229473231501492,
1.44804559906066));
#34062=CARTESIAN_POINT('Ctrl Pts',(5.02476069807077,-0.902005151158387,
1.12142327819778));
#34063=CARTESIAN_POINT('Ctrl Pts',(5.11414214502143,-1.44253731235627,0.453534796061982));
#34064=CARTESIAN_POINT('Ctrl Pts',(5.22630308574295,-1.4458617461083,-0.704791410686178));
#34065=CARTESIAN_POINT('Ctrl Pts',(5.36180677972868,-0.349337730909665,
-1.58269217180053));
#34066=CARTESIAN_POINT('Ctrl Pts',(5.49842670840074,1.02827880679783,-1.26994462762035));
#34067=CARTESIAN_POINT('Ctrl Pts',(5.63636184857256,1.65389902289474,0.0147413000363786));
#34068=CARTESIAN_POINT('Ctrl Pts',(5.76418317065839,1.07983232656629,1.20601509187628));
#34069=CARTESIAN_POINT('Ctrl Pts',(5.88159777082462,-0.0199377183914416,
1.58882970514278));
#34070=CARTESIAN_POINT('Ctrl Pts',(5.98828065981164,-1.01646279733448,1.24276792091335));
#34071=CARTESIAN_POINT('Ctrl Pts',(6.09602860027055,-1.58629611726947,0.339763321778818));
#34072=CARTESIAN_POINT('Ctrl Pts',(6.20490847258959,-1.46716302714867,-0.731395319267634));
#34073=CARTESIAN_POINT('Ctrl Pts',(6.31494726512681,-0.698554879731498,
-1.50380945298764));
#34074=CARTESIAN_POINT('Ctrl Pts',(6.42623832876641,0.396834532462986,-1.62857970257978));
#34075=CARTESIAN_POINT('Ctrl Pts',(6.51995917582357,1.18229401202514,-1.1375069093975));
#34076=CARTESIAN_POINT('Ctrl Pts',(6.59569195310362,1.52939583473763,-0.505043507088318));
#34077=CARTESIAN_POINT('Ctrl Pts',(6.63371330954042,1.58973057564736,-0.154190128191221));
#34078=CARTESIAN_POINT('Ctrl Pts',(6.65276483375079,1.59006621547548,0.0270987442288496));
#34079=CARTESIAN_POINT('Ctrl Pts',(0.201836006562775,1.92995577875298,0.00663072711028962));
#34080=CARTESIAN_POINT('Ctrl Pts',(0.224795078860765,1.9295512977723,0.225102712807887));
#34081=CARTESIAN_POINT('Ctrl Pts',(0.271213486384443,1.85616115643364,0.653502313542884));
#34082=CARTESIAN_POINT('Ctrl Pts',(0.363604583187976,1.43267031234386,1.42506685239735));
#34083=CARTESIAN_POINT('Ctrl Pts',(0.479576972855799,0.463331817377741,
2.03555787261258));
#34084=CARTESIAN_POINT('Ctrl Pts',(0.618629625107766,-0.906182013551074,
1.88150617936703));
#34085=CARTESIAN_POINT('Ctrl Pts',(0.757746114284183,-1.87958474430334,
0.9076648120197));
#34086=CARTESIAN_POINT('Ctrl Pts',(0.896706311574424,-2.03342734252753,
-0.459866228468009));
#34087=CARTESIAN_POINT('Ctrl Pts',(1.03546170358268,-1.30229481563026,-1.62266197721363));
#34088=CARTESIAN_POINT('Ctrl Pts',(1.1738866891073,-0.00771058607069546,
-2.07527455834761));
#34089=CARTESIAN_POINT('Ctrl Pts',(1.29655718944891,1.13725471717341,-1.67217948259824));
#34090=CARTESIAN_POINT('Ctrl Pts',(1.40355524104465,1.77588206025209,-0.868120367571199));
#34091=CARTESIAN_POINT('Ctrl Pts',(1.49500705634901,1.97148816005587,-0.0130330893690973));
#34092=CARTESIAN_POINT('Ctrl Pts',(1.58617102513088,1.77617516983714,0.839207774540849));
#34093=CARTESIAN_POINT('Ctrl Pts',(1.67701884112096,1.23252947154644,1.52155822726773));
#34094=CARTESIAN_POINT('Ctrl Pts',(1.76752485196204,0.451082218560783,1.89514370110071));
#34095=CARTESIAN_POINT('Ctrl Pts',(1.88770765503142,-0.705441630270057,
1.90264440991584));
#34096=CARTESIAN_POINT('Ctrl Pts',(2.03695468071265,-1.9081838550806,0.94032766212397));
#34097=CARTESIAN_POINT('Ctrl Pts',(2.18473095478842,-1.90658288368755,-0.589977958798058));
#34098=CARTESIAN_POINT('Ctrl Pts',(2.30198581617906,-1.19676910050402,-1.46411874702317));
#34099=CARTESIAN_POINT('Ctrl Pts',(2.41857160900784,-0.191636557767527,
-1.95505543786729));
#34100=CARTESIAN_POINT('Ctrl Pts',(2.5629888947828,1.2663632428723,-1.62394356863633));
#34101=CARTESIAN_POINT('Ctrl Pts',(2.73407115542912,2.0270803897522,-0.0201760536951305));
#34102=CARTESIAN_POINT('Ctrl Pts',(2.87468753311021,1.39305244293906,1.28367355357035));
#34103=CARTESIAN_POINT('Ctrl Pts',(2.985961186478,0.424866500577374,1.74094181792175));
#34104=CARTESIAN_POINT('Ctrl Pts',(3.06879765074836,-0.367776933829584,
1.74199341254035));
#34105=CARTESIAN_POINT('Ctrl Pts',(3.15100736921607,-1.0788356648381,1.39845630998696));
#34106=CARTESIAN_POINT('Ctrl Pts',(3.23258126027651,-1.56616872509529,0.786326708824376));
#34107=CARTESIAN_POINT('Ctrl Pts',(3.31351914497578,-1.73765670717964,0.0294003216284019));
#34108=CARTESIAN_POINT('Ctrl Pts',(3.40719584708756,-1.53805092823913,-0.847373922431961));
#34109=CARTESIAN_POINT('Ctrl Pts',(3.51317550457446,-0.79697103399377,-1.58892396461612));
#34110=CARTESIAN_POINT('Ctrl Pts',(3.63093975483762,0.364087451579112,-1.71693586757571));
#34111=CARTESIAN_POINT('Ctrl Pts',(3.74726185074701,1.33676222663195,-1.10142473675384));
#34112=CARTESIAN_POINT('Ctrl Pts',(3.86213882267644,1.71071625332947,-0.0269760307547636));
#34113=CARTESIAN_POINT('Ctrl Pts',(3.97559755033401,1.33734506143431,1.03260709602997));
#34114=CARTESIAN_POINT('Ctrl Pts',(4.08766375246609,0.39658526295041,1.62104472468397));
#34115=CARTESIAN_POINT('Ctrl Pts',(4.19837188466259,-0.692552398864759,
1.49604314345822));
#34116=CARTESIAN_POINT('Ctrl Pts',(4.30776281443248,-1.4569519090562,0.728544173315976));
#34117=CARTESIAN_POINT('Ctrl Pts',(4.41588440940527,-1.57476055190118,-0.335612967324715));
#34118=CARTESIAN_POINT('Ctrl Pts',(4.52279088240793,-1.0098659333688,-1.23091885839333));
#34119=CARTESIAN_POINT('Ctrl Pts',(4.62854271946233,-0.0208637422853108,
-1.57498366840481));
#34120=CARTESIAN_POINT('Ctrl Pts',(4.73320651333447,0.956721615277288,-1.23104232731158));
#34121=CARTESIAN_POINT('Ctrl Pts',(4.83685381440459,1.50113720788295,-0.361046551352442));
#34122=CARTESIAN_POINT('Ctrl Pts',(4.93956680559533,1.38675857073312,0.649275822959622));
#34123=CARTESIAN_POINT('Ctrl Pts',(5.04141762750123,0.672155174078915,1.36176713203313));
#34124=CARTESIAN_POINT('Ctrl Pts',(5.13126818486399,-0.212417836755547,
1.45954591835434));
#34125=CARTESIAN_POINT('Ctrl Pts',(5.20944866403957,-0.885934908127286,
1.13191422290279));
#34126=CARTESIAN_POINT('Ctrl Pts',(5.29843130100065,-1.42368217894501,0.466316024045218));
#34127=CARTESIAN_POINT('Ctrl Pts',(5.40904405233104,-1.42383866211022,-0.676135006079988));
#34128=CARTESIAN_POINT('Ctrl Pts',(5.54102654373605,-0.35328520959894,-1.5282437999679));
#34129=CARTESIAN_POINT('Ctrl Pts',(5.67249721216457,0.971590168067238,-1.22370899227755));
#34130=CARTESIAN_POINT('Ctrl Pts',(5.80369886270088,1.5635297180874,-0.00010031995261808));
#34131=CARTESIAN_POINT('Ctrl Pts',(5.92394544959964,1.02078935752518,1.11925283857749));
#34132=CARTESIAN_POINT('Ctrl Pts',(6.03342516804945,-0.00501638868570453,
1.47478640897076));
#34133=CARTESIAN_POINT('Ctrl Pts',(6.13218887234589,-0.92723326445955,1.15337619506912));
#34134=CARTESIAN_POINT('Ctrl Pts',(6.23127805234855,-1.45037454055268,0.322285760023574));
#34135=CARTESIAN_POINT('Ctrl Pts',(6.33081386970904,-1.34051708598646,-0.656728344800009));
#34136=CARTESIAN_POINT('Ctrl Pts',(6.43084535343457,-0.641085133745283,
-1.35854714858885));
#34137=CARTESIAN_POINT('Ctrl Pts',(6.53157235049208,0.350142317022017,-1.47042556616477));
#34138=CARTESIAN_POINT('Ctrl Pts',(6.61595803451021,1.05760233194793,-1.02813235011111));
#34139=CARTESIAN_POINT('Ctrl Pts',(6.68412403526691,1.36966491076677,-0.458766422246885));
#34140=CARTESIAN_POINT('Ctrl Pts',(6.7181331127701,1.42366222550641,-0.144933967556013));
#34141=CARTESIAN_POINT('Ctrl Pts',(6.73533237399976,1.42396523313032,0.0187292984563378));
#34142=CARTESIAN_POINT('Ctrl Pts',(0.0055986102182942,1.7786917886362,0.0269731300457806));
#34143=CARTESIAN_POINT('Ctrl Pts',(0.0269030153260128,1.77831645872047,
0.229699774553832));
#34144=CARTESIAN_POINT('Ctrl Pts',(0.0697170102000981,1.71067986121277,
0.624862173397813));
#34145=CARTESIAN_POINT('Ctrl Pts',(0.155518742768547,1.31788830620784,1.34153507286603));
#34146=CARTESIAN_POINT('Ctrl Pts',(0.263771619458144,0.413530357430306,
1.91245230228306));
#34147=CARTESIAN_POINT('Ctrl Pts',(0.394742448193518,-0.876433246166832,
1.76940441846535));
#34148=CARTESIAN_POINT('Ctrl Pts',(0.526895266046311,-1.8025697956283,0.845508368090719));
#34149=CARTESIAN_POINT('Ctrl Pts',(0.6600878321834,-1.95199027993901,-0.464994289895076));
#34150=CARTESIAN_POINT('Ctrl Pts',(0.794281538807695,-1.24660356207781,
-1.59065630973919));
#34151=CARTESIAN_POINT('Ctrl Pts',(0.929381540394946,0.0161873708636046,
-2.03437466461124));
#34152=CARTESIAN_POINT('Ctrl Pts',(1.05020992338902,1.14459879547428,-1.63901960444341));
#34153=CARTESIAN_POINT('Ctrl Pts',(1.1564113362939,1.77908325177254,-0.841350702215082));
#34154=CARTESIAN_POINT('Ctrl Pts',(1.24774422943565,1.97499565916099,0.0124643607619269));
#34155=CARTESIAN_POINT('Ctrl Pts',(1.33935066447099,1.77932241292938,0.868971342433958));
#34156=CARTESIAN_POINT('Ctrl Pts',(1.43120343117607,1.23018382091282,1.55925189286057));
#34157=CARTESIAN_POINT('Ctrl Pts',(1.52327258476988,0.435406173219395,1.93975522009938));
#34158=CARTESIAN_POINT('Ctrl Pts',(1.64628334757985,-0.747955935764237,
1.94844299211941));
#34159=CARTESIAN_POINT('Ctrl Pts',(1.80043942830411,-1.99282994775571,0.957661401566267));
#34160=CARTESIAN_POINT('Ctrl Pts',(1.95492260956612,-1.99542728549998,-0.64185356411705));
#34161=CARTESIAN_POINT('Ctrl Pts',(2.07857944637526,-1.2473256436638,-1.5645532630108));
#34162=CARTESIAN_POINT('Ctrl Pts',(2.20224026315262,-0.181801586351347,
-2.08583346026664));
#34163=CARTESIAN_POINT('Ctrl Pts',(2.35676056686682,1.37874519474033,-1.73564260477601));
#34164=CARTESIAN_POINT('Ctrl Pts',(2.54182526832312,2.20609106907775,-0.00268827228171362));
#34165=CARTESIAN_POINT('Ctrl Pts',(2.69555119442166,1.51605336872507,1.42417233727536));
#34166=CARTESIAN_POINT('Ctrl Pts',(2.81811658390143,0.449775260975512,1.92865218693433));
#34167=CARTESIAN_POINT('Ctrl Pts',(2.90980425579794,-0.427472809728478,
1.93018337506389));
#34168=CARTESIAN_POINT('Ctrl Pts',(3.0012257313044,-1.21838376850936,1.54862371335145));
#34169=CARTESIAN_POINT('Ctrl Pts',(3.09235597402077,-1.76311410577726,0.865082768968332));
#34170=CARTESIAN_POINT('Ctrl Pts',(3.18316203145471,-1.95590236528654,0.0159781933622966));
#34171=CARTESIAN_POINT('Ctrl Pts',(3.28869781156922,-1.73151158460335,-0.971832032847293));
#34172=CARTESIAN_POINT('Ctrl Pts',(3.40869099291695,-0.893323402037981,
-1.81213480121132));
#34173=CARTESIAN_POINT('Ctrl Pts',(3.5427667337023,0.428303253574616,-1.95909052352705));
#34174=CARTESIAN_POINT('Ctrl Pts',(3.67583348666243,1.54154498477032,-1.25584048760503));
#34175=CARTESIAN_POINT('Ctrl Pts',(3.80783173039662,1.97204661692226,-0.0216508987713537));
#34176=CARTESIAN_POINT('Ctrl Pts',(3.93868718175276,1.5421657385633,1.20058177185902));
#34177=CARTESIAN_POINT('Ctrl Pts',(4.06833893810746,0.454165564969672,1.88182985373663));
#34178=CARTESIAN_POINT('Ctrl Pts',(4.19673100805262,-0.808925769374989,
1.73731835455084));
#34179=CARTESIAN_POINT('Ctrl Pts',(4.32381422461611,-1.6971140366654,0.845943606081325));
#34180=CARTESIAN_POINT('Ctrl Pts',(4.44954593492418,-1.83423268382295,-0.391455693145508));
#34181=CARTESIAN_POINT('Ctrl Pts',(4.57389042061536,-1.17720068138488,-1.43272620490813));
#34182=CARTESIAN_POINT('Ctrl Pts',(4.69681904943983,-0.0275512378076592,
-1.83246320358028));
#34183=CARTESIAN_POINT('Ctrl Pts',(4.81831031197903,1.10702608934609,-1.43289530427454));
#34184=CARTESIAN_POINT('Ctrl Pts',(4.9383507013174,1.73706127318637,-0.425069901136755));
#34185=CARTESIAN_POINT('Ctrl Pts',(5.05692960886477,1.60431828004724,0.741229170655166));
#34186=CARTESIAN_POINT('Ctrl Pts',(5.17405567081681,0.78196805313534,1.55992384717266));
#34187=CARTESIAN_POINT('Ctrl Pts',(5.27687879209034,-0.230347348735859,
1.67087959864774));
#34188=CARTESIAN_POINT('Ctrl Pts',(5.36591877038285,-0.997165099457179,
1.29747944846882));
#34189=CARTESIAN_POINT('Ctrl Pts',(5.46683882163731,-1.60675724871016,0.542112054460348));
#34190=CARTESIAN_POINT('Ctrl Pts',(5.59143208581872,-1.60417349359218,-0.744753029658688));
#34191=CARTESIAN_POINT('Ctrl Pts',(5.7385327841038,-0.408499051200149,-1.69141896776007));
#34192=CARTESIAN_POINT('Ctrl Pts',(5.883324066422,1.04964479963234,-1.35191858333315));
#34193=CARTESIAN_POINT('Ctrl Pts',(6.02592910385855,1.68891108077235,-0.0198425009263074));
#34194=CARTESIAN_POINT('Ctrl Pts',(6.15477896868988,1.10345053670017,1.17755753597987));
#34195=CARTESIAN_POINT('Ctrl Pts',(6.27054089751149,0.0181739231631492,
1.55116490184665));
#34196=CARTESIAN_POINT('Ctrl Pts',(6.37374590914519,-0.944877441319298,
1.21343625499497));
#34197=CARTESIAN_POINT('Ctrl Pts',(6.47603956445423,-1.48313972011788,0.354292762592425));
#34198=CARTESIAN_POINT('Ctrl Pts',(6.57752721567845,-1.36903420817986,-0.643670764365519));
#34199=CARTESIAN_POINT('Ctrl Pts',(6.67824768359502,-0.663252374784276,
-1.34885741154892));
#34200=CARTESIAN_POINT('Ctrl Pts',(6.77839723147235,0.322508461880067,-1.45796924039956));
#34201=CARTESIAN_POINT('Ctrl Pts',(6.86124765395301,1.01625734071238,-1.02232645390806));
#34202=CARTESIAN_POINT('Ctrl Pts',(6.92756787351227,1.31944073792609,-0.468256814773046));
#34203=CARTESIAN_POINT('Ctrl Pts',(6.96040226429529,1.37148079685521,-0.165228975162103));
#34204=CARTESIAN_POINT('Ctrl Pts',(6.97707472275653,1.3717745235424,-0.00657861409212436));
#34205=CARTESIAN_POINT('Ctrl Pts',(0.00161515851542798,1.53044829317965,
0.0269321480552476));
#34206=CARTESIAN_POINT('Ctrl Pts',(0.0201220759100287,1.53012224794576,
0.20303869712926));
#34207=CARTESIAN_POINT('Ctrl Pts',(0.0568934829114929,1.47197746737321,
0.542427739520397));
#34208=CARTESIAN_POINT('Ctrl Pts',(0.131095753839526,1.13271443757942,1.16232575285471));
#34209=CARTESIAN_POINT('Ctrl Pts',(0.224621021627344,0.35091150368134,1.65551025424783));
#34210=CARTESIAN_POINT('Ctrl Pts',(0.338286873126993,-0.768313442313391,
1.53243149360112));
#34211=CARTESIAN_POINT('Ctrl Pts',(0.453361445182077,-1.57547718717538,
0.728139909528747));
#34212=CARTESIAN_POINT('Ctrl Pts',(0.569884598800981,-1.70710757953583,
-0.418100970988217));
#34213=CARTESIAN_POINT('Ctrl Pts',(0.687857467706789,-1.08784745868724,
-1.40832549057182));
#34214=CARTESIAN_POINT('Ctrl Pts',(0.807288840150634,0.0280726252692547,
-1.80167751441015));
#34215=CARTESIAN_POINT('Ctrl Pts',(0.914740219816513,1.03198965030329,-1.45112979405465));
#34216=CARTESIAN_POINT('Ctrl Pts',(1.00969670875881,1.59968282864761,-0.738184106724425));
#34217=CARTESIAN_POINT('Ctrl Pts',(1.09172273732053,1.77602714402117,0.0285405148911991));
#34218=CARTESIAN_POINT('Ctrl Pts',(1.17437872066553,1.59987524911727,0.801458775626711));
#34219=CARTESIAN_POINT('Ctrl Pts',(1.25765544748547,1.10238644594154,1.4275960011703));
#34220=CARTESIAN_POINT('Ctrl Pts',(1.34154470845672,0.378319431930998,1.7746505260415));
#34221=CARTESIAN_POINT('Ctrl Pts',(1.45419701031386,-0.705136228348483,
1.78339235323209));
#34222=CARTESIAN_POINT('Ctrl Pts',(1.59648741121626,-1.8563330628512,0.871461571340324));
#34223=CARTESIAN_POINT('Ctrl Pts',(1.74064586963647,-1.86249944592916,-0.621030337744628));
#34224=CARTESIAN_POINT('Ctrl Pts',(1.85702935773388,-1.15881384850636,-1.4902952011907));
#34225=CARTESIAN_POINT('Ctrl Pts',(1.97409322998411,-0.15066510931235,-1.98428777225483));
#34226=CARTESIAN_POINT('Ctrl Pts',(2.12163828274568,1.34022641380533,-1.65398375350995));
#34227=CARTESIAN_POINT('Ctrl Pts',(2.30048850270571,2.14467296000503,0.0187913828637551));
#34228=CARTESIAN_POINT('Ctrl Pts',(2.45086488774202,1.47323008289345,1.4163874062059));
#34229=CARTESIAN_POINT('Ctrl Pts',(2.57186497454107,0.420695575966319,1.91549206070169));
#34230=CARTESIAN_POINT('Ctrl Pts',(2.66293836951461,-0.450677600870363,
1.91750519917846));
#34231=CARTESIAN_POINT('Ctrl Pts',(2.7543083824095,-1.24144775215012,1.53674405551446));
#34232=CARTESIAN_POINT('Ctrl Pts',(2.845945416743,-1.78973088627105,0.849726749694565));
#34233=CARTESIAN_POINT('Ctrl Pts',(2.93782583740514,-1.98537059820214,-0.00933625461138338));
#34234=CARTESIAN_POINT('Ctrl Pts',(3.0452661736348,-1.75766233264543,-1.01511590115231));
#34235=CARTESIAN_POINT('Ctrl Pts',(3.16835592453166,-0.899160965219046,
-1.87833647594073));
#34236=CARTESIAN_POINT('Ctrl Pts',(3.30713426793985,0.468701930885861,-2.03267167226986));
#34237=CARTESIAN_POINT('Ctrl Pts',(3.44612725137011,1.63270311246182,-1.29975466142584));
#34238=CARTESIAN_POINT('Ctrl Pts',(3.58521702248767,2.08828439185582,0.000128743541493508));
#34239=CARTESIAN_POINT('Ctrl Pts',(3.72430585843795,1.63321566517972,1.30001690797893));
#34240=CARTESIAN_POINT('Ctrl Pts',(3.86328811026007,0.467872078525812,2.03198524404679));
#34241=CARTESIAN_POINT('Ctrl Pts',(4.00206055629492,-0.897638539459245,
1.87766260277105));
#34242=CARTESIAN_POINT('Ctrl Pts',(4.14052047602126,-1.86669284198261,0.907716764412239));
#34243=CARTESIAN_POINT('Ctrl Pts',(4.27856708575799,-2.0189887304933,-0.450770285803224));
#34244=CARTESIAN_POINT('Ctrl Pts',(4.41610166348544,-1.29362389666168,-1.60345254256816));
#34245=CARTESIAN_POINT('Ctrl Pts',(4.55302789008076,-0.0135058866939321,
-2.050212795458));
#34246=CARTESIAN_POINT('Ctrl Pts',(4.68925261674667,1.25922415346523,-1.60354209644131));
#34247=CARTESIAN_POINT('Ctrl Pts',(4.82468558038221,1.9712326392338,-0.467118840728988));
#34248=CARTESIAN_POINT('Ctrl Pts',(4.95924592020433,1.82182897712141,0.856515477717086));
#34249=CARTESIAN_POINT('Ctrl Pts',(5.09284396200303,0.884552093304522,1.79121367849672));
#34250=CARTESIAN_POINT('Ctrl Pts',(5.21068038662158,-0.275570397721873,
1.91923933957688));
#34251=CARTESIAN_POINT('Ctrl Pts',(5.31307309209999,-1.15755384723355,1.49002958567083));
#34252=CARTESIAN_POINT('Ctrl Pts',(5.42941292464469,-1.86054864392746,0.619529830873306));
#34253=CARTESIAN_POINT('Ctrl Pts',(5.57351539554265,-1.85877020130954,-0.868886341085341));
#34254=CARTESIAN_POINT('Ctrl Pts',(5.74418971119599,-0.472056341979532,
-1.96814250186018));
#34255=CARTESIAN_POINT('Ctrl Pts',(5.91250379993996,1.22319597970524,-1.5739132963462));
#34256=CARTESIAN_POINT('Ctrl Pts',(6.07836620391931,1.96669257276546,-0.0244705791669788));
#34257=CARTESIAN_POINT('Ctrl Pts',(6.22809494634827,1.28580890149433,1.36676280853955));
#34258=CARTESIAN_POINT('Ctrl Pts',(6.36234254672962,0.0270514125726567,
1.79951128756652));
#34259=CARTESIAN_POINT('Ctrl Pts',(6.48171218482806,-1.08665979377014,1.40829938442376));
#34260=CARTESIAN_POINT('Ctrl Pts',(6.59962381806671,-1.70640593150187,0.417640574653327));
#34261=CARTESIAN_POINT('Ctrl Pts',(6.71608583977231,-1.57451406593522,-0.727604326553729));
#34262=CARTESIAN_POINT('Ctrl Pts',(6.83109988901939,-0.767942536703866,
-1.53166897248179));
#34263=CARTESIAN_POINT('Ctrl Pts',(6.94470644964824,0.350764911141124,-1.65459943602436));
#34264=CARTESIAN_POINT('Ctrl Pts',(7.03818284450952,1.13212881810176,-1.16171427974159));
#34265=CARTESIAN_POINT('Ctrl Pts',(7.1123475034697,1.47122577126917,-0.542122479375375));
#34266=CARTESIAN_POINT('Ctrl Pts',(7.14909956085597,1.52933816287858,-0.202914044278201));
#34267=CARTESIAN_POINT('Ctrl Pts',(7.16759750918473,1.52966405009522,-0.0268928421120539));
#34268=CARTESIAN_POINT('Ctrl Pts',(0.191650118418653,1.37200316952796,0.00666815673193312));
#34269=CARTESIAN_POINT('Ctrl Pts',(0.208325719758175,1.37170938746674,0.165348424386552));
#34270=CARTESIAN_POINT('Ctrl Pts',(0.241166543218968,1.31965892482236,0.468436764487971));
#34271=CARTESIAN_POINT('Ctrl Pts',(0.307500414610168,1.01641958147785,1.0226151319287));
#34272=CARTESIAN_POINT('Ctrl Pts',(0.390369372912809,0.322487480659442,
1.45839154679416));
#34273=CARTESIAN_POINT('Ctrl Pts',(0.490545507503801,-0.663481834066145,
1.34918217829499));
#34274=CARTESIAN_POINT('Ctrl Pts',(0.591296831845559,-1.36962537389197,
0.643945208842946));
#34275=CARTESIAN_POINT('Ctrl Pts',(0.692819022950002,-1.4834868198206,-0.354693992611235));
#34276=CARTESIAN_POINT('Ctrl Pts',(0.79515128124215,-0.945721582226587,
-1.21334885843603));
#34277=CARTESIAN_POINT('Ctrl Pts',(0.898397805393483,0.019124050649053,
-1.55286223755737));
#34278=CARTESIAN_POINT('Ctrl Pts',(0.991048529453213,0.884620402844577,
-1.25029479050423));
#34279=CARTESIAN_POINT('Ctrl Pts',(1.07280457269834,1.37332023443167,-0.636418491153494));
#34280=CARTESIAN_POINT('Ctrl Pts',(1.14337435396381,1.52497778900527,0.0232193216955604));
#34281=CARTESIAN_POINT('Ctrl Pts',(1.21445487160599,1.37347475326106,0.687882348496639));
#34282=CARTESIAN_POINT('Ctrl Pts',(1.28606621168212,0.945692747518926,1.22628909211129));
#34283=CARTESIAN_POINT('Ctrl Pts',(1.35822394446807,0.322887605036237,1.52484062894975));
#34284=CARTESIAN_POINT('Ctrl Pts',(1.45518726216361,-0.609556983176929,
1.53241846122719));
#34285=CARTESIAN_POINT('Ctrl Pts',(1.57783368086597,-1.60225845024684,0.746967726957822));
#34286=CARTESIAN_POINT('Ctrl Pts',(1.70249589452176,-1.60863592636691,-0.543521601599762));
#34287=CARTESIAN_POINT('Ctrl Pts',(1.80347019036147,-0.998354974154592,
-1.29794080715334));
#34288=CARTESIAN_POINT('Ctrl Pts',(1.90528174786493,-0.12178238469645,-1.72773866254481));
#34289=CARTESIAN_POINT('Ctrl Pts',(2.03415464227018,1.18048402935804,-1.44105642428614));
#34290=CARTESIAN_POINT('Ctrl Pts',(2.19137194686348,1.89005998100612,0.0282102837295534));
#34291=CARTESIAN_POINT('Ctrl Pts',(2.32454795335086,1.29747855460094,1.26686334860849));
#34292=CARTESIAN_POINT('Ctrl Pts',(2.43238000253166,0.359684880651055,1.71226358790709));
#34293=CARTESIAN_POINT('Ctrl Pts',(2.51389508088681,-0.420163686752707,
1.71436684276211));
#34294=CARTESIAN_POINT('Ctrl Pts',(2.59604473430107,-1.13126882064223,1.37245282944764));
#34295=CARTESIAN_POINT('Ctrl Pts',(2.67882608336087,-1.62685859758749,0.752138485726358));
#34296=CARTESIAN_POINT('Ctrl Pts',(2.76222187864817,-1.80485064039527,-0.0274796911837139));
#34297=CARTESIAN_POINT('Ctrl Pts',(2.86022959910713,-1.59768976513308,-0.944989781542403));
#34298=CARTESIAN_POINT('Ctrl Pts',(2.97324187521099,-0.810607665017154,
-1.73843407949934));
#34299=CARTESIAN_POINT('Ctrl Pts',(3.1016972315778,0.455113169607269,-1.88310324228184));
#34300=CARTESIAN_POINT('Ctrl Pts',(3.23139431556386,1.5422393319403,-1.20073842659454));
#34301=CARTESIAN_POINT('Ctrl Pts',(3.3623017082119,1.97273947585015,0.0219070491777476));
#34302=CARTESIAN_POINT('Ctrl Pts',(3.49434572163654,1.54259771177146,1.25649542936377));
#34303=CARTESIAN_POINT('Ctrl Pts',(3.6274603391642,0.427609280977633,1.95918845230357));
#34304=CARTESIAN_POINT('Ctrl Pts',(3.76157159803446,-0.89215437286064,1.81208933337819));
#34305=CARTESIAN_POINT('Ctrl Pts',(3.89660124235199,-1.83859312657177,0.867715935336504));
#34306=CARTESIAN_POINT('Ctrl Pts',(4.03246592923656,-1.99055769088599,-0.468958872232718));
#34307=CARTESIAN_POINT('Ctrl Pts',(4.16907822980912,-1.27190965259628,-1.61495361257738));
#34308=CARTESIAN_POINT('Ctrl Pts',(4.30634680696854,0.0106137187745297,
-2.06480696177015));
#34309=CARTESIAN_POINT('Ctrl Pts',(4.44417666851365,1.29894786746045,-1.61491946025705));
#34310=CARTESIAN_POINT('Ctrl Pts',(4.58247097086598,2.02777293713842,-0.455689806908409));
#34311=CARTESIAN_POINT('Ctrl Pts',(4.72112199455802,1.87589664300924,0.908314574073854));
#34312=CARTESIAN_POINT('Ctrl Pts',(4.86004315540616,0.902897634535989,1.88170990575402));
#34313=CARTESIAN_POINT('Ctrl Pts',(4.98366759096385,-0.314015698055534,
2.01785190496137));
#34314=CARTESIAN_POINT('Ctrl Pts',(5.09187133849345,-1.24637851798351,1.56480044764036));
#34315=CARTESIAN_POINT('Ctrl Pts',(5.21552467151859,-1.99407016576495,0.640432896817704));
#34316=CARTESIAN_POINT('Ctrl Pts',(5.3699969526124,-1.99604585088204,-0.954985827792077));
#34317=CARTESIAN_POINT('Ctrl Pts',(5.55496725528798,-0.496223154682238,
-2.14999595683691));
#34318=CARTESIAN_POINT('Ctrl Pts',(5.73929698552342,1.36136728950175,-1.7225381487768));
#34319=CARTESIAN_POINT('Ctrl Pts',(5.92275132000792,2.18746307299438,-0.0106556007638544));
#34320=CARTESIAN_POINT('Ctrl Pts',(6.08990782660862,1.43044508811081,1.5441079994423));
#34321=CARTESIAN_POINT('Ctrl Pts',(6.24090189886119,0.0150536285141992,
2.03247023467283));
#34322=CARTESIAN_POINT('Ctrl Pts',(6.37596384346278,-1.245467488101,1.59099367856498));
#34323=CARTESIAN_POINT('Ctrl Pts',(6.51011494443758,-1.95157823607613,0.464639836930734));
#34324=CARTESIAN_POINT('Ctrl Pts',(6.64326231244002,-1.80182018279085,-0.844992615596695));
#34325=CARTESIAN_POINT('Ctrl Pts',(6.77536637951215,-0.876213641136945,
-1.76877236414733));
#34326=CARTESIAN_POINT('Ctrl Pts',(6.90628636007342,0.413337672718451,-1.91167105187073));
#34327=CARTESIAN_POINT('Ctrl Pts',(7.01449296705847,1.317278997971,-1.34103733354681));
#34328=CARTESIAN_POINT('Ctrl Pts',(7.10025971255133,1.70991664822488,-0.624645108920693));
#34329=CARTESIAN_POINT('Ctrl Pts',(7.14305493470294,1.77751904014347,-0.229658083660462));
#34330=CARTESIAN_POINT('Ctrl Pts',(7.16435095364275,1.77789422231039,-0.0270112393448257));
#34331=CARTESIAN_POINT('Ctrl Pts',(0.433579734615651,1.42338264829905,-0.0186609375666422));
#34332=CARTESIAN_POINT('Ctrl Pts',(0.45077175068432,1.42307976831204,0.144933385405884));
#34333=CARTESIAN_POINT('Ctrl Pts',(0.484766255202398,1.36910205511848,0.458630441946588));
#34334=CARTESIAN_POINT('Ctrl Pts',(0.552904217423861,1.05717509657061,1.02775607980824));
#34335=CARTESIAN_POINT('Ctrl Pts',(0.637261343794741,0.349940230409029,
1.46993737614911));
#34336=CARTESIAN_POINT('Ctrl Pts',(0.737955078347263,-0.64090291216559,
1.35804969385912));
#34337=CARTESIAN_POINT('Ctrl Pts',(0.837958305020876,-1.34029379299783,
0.656595041185004));
#34338=CARTESIAN_POINT('Ctrl Pts',(0.937469751658734,-1.44986143925427,
-0.322474352691997));
#34339=CARTESIAN_POINT('Ctrl Pts',(1.03653768857201,-0.927532143269398,
-1.15270388821428));
#34340=CARTESIAN_POINT('Ctrl Pts',(1.13528664206825,-0.00406063929822328,
-1.47553624283577));
#34341=CARTESIAN_POINT('Ctrl Pts',(1.22285503142353,0.813435828702286,-1.18804460975032));
#34342=CARTESIAN_POINT('Ctrl Pts',(1.2994077250104,1.27049736626634,-0.612887311395251));
#34343=CARTESIAN_POINT('Ctrl Pts',(1.36499674892347,1.41100310001544,0.00035353166708084));
#34344=CARTESIAN_POINT('Ctrl Pts',(1.43059568312704,1.27070020510333,0.61366388234097));
#34345=CARTESIAN_POINT('Ctrl Pts',(1.4962312545865,0.878209084856175,1.10687935212739));
#34346=CARTESIAN_POINT('Ctrl Pts',(1.56193801594905,0.310932069106502,1.37839912120734));
#34347=CARTESIAN_POINT('Ctrl Pts',(1.64967414989946,-0.53309404837248,1.38454132805412));
#34348=CARTESIAN_POINT('Ctrl Pts',(1.75967689190248,-1.42179124988727,0.677917697927037));
#34349=CARTESIAN_POINT('Ctrl Pts',(1.87030374837707,-1.42492338598861,-0.467528578572644));
#34350=CARTESIAN_POINT('Ctrl Pts',(1.95930615128506,-0.886719411403927,
-1.13212549488085));
#34351=CARTESIAN_POINT('Ctrl Pts',(2.04868501593063,-0.116842483376934,
-1.50916256492749));
#34352=CARTESIAN_POINT('Ctrl Pts',(2.16113597918497,1.01949045845296,-1.25718641848022));
#34353=CARTESIAN_POINT('Ctrl Pts',(2.29753653972427,1.63359955754855,0.0182741116564148));
#34354=CARTESIAN_POINT('Ctrl Pts',(2.41255997285096,1.12092326938844,1.08784129807883));
#34355=CARTESIAN_POINT('Ctrl Pts',(2.50548250553227,0.312692840718015,1.47156942514894));
#34356=CARTESIAN_POINT('Ctrl Pts',(2.5756478252876,-0.358700517462746,1.47334788294029));
#34357=CARTESIAN_POINT('Ctrl Pts',(2.64631010793517,-0.970420591352287,
1.17915861370463));
#34358=CARTESIAN_POINT('Ctrl Pts',(2.71748033839573,-1.39658058337222,0.645750906017974));
#34359=CARTESIAN_POINT('Ctrl Pts',(2.78919511691523,-1.54965148821638,-0.0247331123591614));
#34360=CARTESIAN_POINT('Ctrl Pts',(2.87350305966914,-1.3714855406497,-0.814073759711593));
#34361=CARTESIAN_POINT('Ctrl Pts',(2.97078939013895,-0.693974426765108,
-1.4973274317204));
#34362=CARTESIAN_POINT('Ctrl Pts',(3.08153687990464,0.39749474778564,-1.62249875077181));
#34363=CARTESIAN_POINT('Ctrl Pts',(3.1936745402062,1.33779004137835,-1.03288036662484));
#34364=CARTESIAN_POINT('Ctrl Pts',(3.30718845046989,1.71177951199544,0.0272883049770704));
#34365=CARTESIAN_POINT('Ctrl Pts',(3.42212730901466,1.33803574566457,1.10238120232907));
#34366=CARTESIAN_POINT('Ctrl Pts',(3.538506378401,0.363549106704547,1.71759100272943));
#34367=CARTESIAN_POINT('Ctrl Pts',(3.65633855270862,-0.796304462599152,
1.58934728787291));
#34368=CARTESIAN_POINT('Ctrl Pts',(3.77562775390538,-1.63334363828854,0.755741510627042));
#34369=CARTESIAN_POINT('Ctrl Pts',(3.89637125571665,-1.76965210710189,-0.432192879453737));
#34370=CARTESIAN_POINT('Ctrl Pts',(4.01855873411348,-1.12794076480263,-1.45803741696457));
#34371=CARTESIAN_POINT('Ctrl Pts',(4.14217229917805,0.0266723610995444,
-1.86455751754551));
#34372=CARTESIAN_POINT('Ctrl Pts',(4.26718715875757,1.19587440059458,-1.45789650543289));
#34373=CARTESIAN_POINT('Ctrl Pts',(4.39356916365005,1.86336783373069,-0.399233077619641));
#34374=CARTESIAN_POINT('Ctrl Pts',(4.5212929060358,1.72515502607219,0.857488857248103));
#34375=CARTESIAN_POINT('Ctrl Pts',(4.65028582120944,0.822837389786965,1.76269613439977));
#34376=CARTESIAN_POINT('Ctrl Pts',(4.76604443107118,-0.316629397701036,
1.89185367539892));
#34377=CARTESIAN_POINT('Ctrl Pts',(4.86809768231334,-1.1964095449954,1.46496928641178));
#34378=CARTESIAN_POINT('Ctrl Pts',(4.98539825189974,-1.90620592827337,0.588811917862644));
#34379=CARTESIAN_POINT('Ctrl Pts',(5.1332295071313,-1.91202735868246,-0.938044171791657));
#34380=CARTESIAN_POINT('Ctrl Pts',(5.31238298578506,-0.462560121218143,
-2.09951488460516));
#34381=CARTESIAN_POINT('Ctrl Pts',(5.49310436300435,1.35991583640525,-1.68538171905435));
#34382=CARTESIAN_POINT('Ctrl Pts',(5.67518902663768,2.18456796062644,0.0113588410607889));
#34383=CARTESIAN_POINT('Ctrl Pts',(5.84314793625201,1.42809693145233,1.57583744405794));
#34384=CARTESIAN_POINT('Ctrl Pts',(5.99651346043047,-0.00890518390018798,
2.07429703179719));
#34385=CARTESIAN_POINT('Ctrl Pts',(6.13495786102797,-1.30163918905444,1.6236443878012));
#34386=CARTESIAN_POINT('Ctrl Pts',(6.27372909181613,-2.03382659165114,0.459724741300774));
#34387=CARTESIAN_POINT('Ctrl Pts',(6.41269993312306,-1.87954606508905,-0.907477856997402));
#34388=CARTESIAN_POINT('Ctrl Pts',(6.55182430461631,-0.906300332924981,
-1.88153117457102));
#34389=CARTESIAN_POINT('Ctrl Pts',(6.69087755354555,0.463291981836397,-2.03547998152785));
#34390=CARTESIAN_POINT('Ctrl Pts',(6.8068530207987,1.43257691496249,-1.42501755139953));
#34391=CARTESIAN_POINT('Ctrl Pts',(6.89923554548022,1.85603723916337,-0.653520444359812));
#34392=CARTESIAN_POINT('Ctrl Pts',(6.94565012946822,1.92942310320324,-0.225166386510263));
#34393=CARTESIAN_POINT('Ctrl Pts',(6.96860631615056,1.92982753334055,-0.00672185930328364));
#34394=CARTESIAN_POINT('Ctrl Pts',(0.507274282535025,1.57083221824462,-0.0261324580079617));
#34395=CARTESIAN_POINT('Ctrl Pts',(0.526112754645697,1.57050033185239,0.153129071208421));
#34396=CARTESIAN_POINT('Ctrl Pts',(0.563671099889176,1.51089822523919,0.499712748256306));
#34397=CARTESIAN_POINT('Ctrl Pts',(0.638531587307084,1.16784235604667,1.12489642057377));
#34398=CARTESIAN_POINT('Ctrl Pts',(0.731169346030264,0.391386187333621,
1.61031900017172));
#34399=CARTESIAN_POINT('Ctrl Pts',(0.841237656753425,-0.691876171660509,
1.48695593269843));
#34400=CARTESIAN_POINT('Ctrl Pts',(0.950117270175318,-1.45259978153303,
0.722851743027934));
#34401=CARTESIAN_POINT('Ctrl Pts',(1.05791430831992,-1.57031827941192,-0.337921120658705));
#34402=CARTESIAN_POINT('Ctrl Pts',(1.16466136624435,-1.00664473279018,-1.23180991269817));
#34403=CARTESIAN_POINT('Ctrl Pts',(1.27042439012675,-0.0172220148914788,
-1.5764787034829));
#34404=CARTESIAN_POINT('Ctrl Pts',(1.36363143937566,0.852328804108645,-1.26948855586366));
#34405=CARTESIAN_POINT('Ctrl Pts',(1.44462089157926,1.33552310991331,-0.660772156033481));
#34406=CARTESIAN_POINT('Ctrl Pts',(1.51369502886818,1.48307233184017,-0.0149411033225211));
#34407=CARTESIAN_POINT('Ctrl Pts',(1.58243335031582,1.33571785928905,0.627597621853533));
#34408=CARTESIAN_POINT('Ctrl Pts',(1.65086776854819,0.926180438835773,1.14147824220308));
#34409=CARTESIAN_POINT('Ctrl Pts',(1.71901564079579,0.337798744691098,1.42277664606786));
#34410=CARTESIAN_POINT('Ctrl Pts',(1.80954699166651,-0.533138243710397,
1.42838884196275));
#34411=CARTESIAN_POINT('Ctrl Pts',(1.92211699882143,-1.44076854634821,0.703312487395003));
#34412=CARTESIAN_POINT('Ctrl Pts',(2.03410697282657,-1.44096567761035,-0.45603039345914));
#34413=CARTESIAN_POINT('Ctrl Pts',(2.12343975147708,-0.900622955850315,
-1.1223056389964));
#34414=CARTESIAN_POINT('Ctrl Pts',(2.21262722357295,-0.132081188978774,
-1.49810670491376));
#34415=CARTESIAN_POINT('Ctrl Pts',(2.32400115347409,0.99212176527143,-1.24571725700378));
#34416=CARTESIAN_POINT('Ctrl Pts',(2.45753819177609,1.58991663374091,0.00400964696824968));
#34417=CARTESIAN_POINT('Ctrl Pts',(2.56896324607187,1.0911031110618,1.03867404971372));
#34418=CARTESIAN_POINT('Ctrl Pts',(2.65830689011116,0.314148482822285,1.40686816583826));
#34419=CARTESIAN_POINT('Ctrl Pts',(2.72544249781257,-0.328068046776882,
1.40825091301288));
#34420=CARTESIAN_POINT('Ctrl Pts',(2.79272924072257,-0.910251615434656,
1.12786562955998));
#34421=CARTESIAN_POINT('Ctrl Pts',(2.86020818788873,-1.31386839710613,0.622124005734457));
#34422=CARTESIAN_POINT('Ctrl Pts',(2.92787301289815,-1.45800869363228,-0.0104270331006981));
#34423=CARTESIAN_POINT('Ctrl Pts',(3.00708815442165,-1.29025655858587,-0.751868478198773));
#34424=CARTESIAN_POINT('Ctrl Pts',(3.09806652405742,-0.656258052591304,
-1.39010016384697));
#34425=CARTESIAN_POINT('Ctrl Pts',(3.20112002170027,0.358888315027333,-1.50555498910911));
#34426=CARTESIAN_POINT('Ctrl Pts',(3.30486699671298,1.22824795529413,-0.959553219448269));
#34427=CARTESIAN_POINT('Ctrl Pts',(3.40947097081598,1.57205004825354,0.0172505142157691));
#34428=CARTESIAN_POINT('Ctrl Pts',(3.51496482062722,1.22855626968513,1.00343097025568));
#34429=CARTESIAN_POINT('Ctrl Pts',(3.62142414278527,0.337170590068482,1.56556264385462));
#34430=CARTESIAN_POINT('Ctrl Pts',(3.7289101906844,-0.72044261482484,1.44818418374162));
#34431=CARTESIAN_POINT('Ctrl Pts',(3.83748189048483,-1.48179526817998,0.689478939216293));
#34432=CARTESIAN_POINT('Ctrl Pts',(3.94719105937069,-1.60536811159166,-0.389593160174116));
#34433=CARTESIAN_POINT('Ctrl Pts',(4.05808411613347,-1.02302204204489,-1.3202678117195));
#34434=CARTESIAN_POINT('Ctrl Pts',(4.17020177333295,0.023945317461627,-1.68883397376188));
#34435=CARTESIAN_POINT('Ctrl Pts',(4.28357766789648,1.08402787750074,-1.32017808730271));
#34436=CARTESIAN_POINT('Ctrl Pts',(4.39824273901555,1.68964083833592,-0.360000126936474));
#34437=CARTESIAN_POINT('Ctrl Pts',(4.51419461860112,1.56435375572891,0.780776691995831));
#34438=CARTESIAN_POINT('Ctrl Pts',(4.63149231723297,0.744360778919685,1.60396130772566));
#34439=CARTESIAN_POINT('Ctrl Pts',(4.73693160879815,-0.293325697447064,
1.72194634915242));
#34440=CARTESIAN_POINT('Ctrl Pts',(4.83004564060015,-1.09603579295444,1.3326447194401));
#34441=CARTESIAN_POINT('Ctrl Pts',(4.93724867578556,-1.74478074698819,0.532228279741075));
#34442=CARTESIAN_POINT('Ctrl Pts',(5.0727192263256,-1.75135757443499,-0.866786972823142));
#34443=CARTESIAN_POINT('Ctrl Pts',(5.2375920787962,-0.418735016597171,-1.93699754149329));
#34444=CARTESIAN_POINT('Ctrl Pts',(5.40471142470201,1.26692786505107,-1.55606606404468));
#34445=CARTESIAN_POINT('Ctrl Pts',(5.57399875094415,2.03565424341948,0.0202999121532512));
#34446=CARTESIAN_POINT('Ctrl Pts',(5.73107580726873,1.33028224859866,1.48442877087329));
#34447=CARTESIAN_POINT('Ctrl Pts',(5.87529457722589,-0.0207131719272176,
1.95442357858293));
#34448=CARTESIAN_POINT('Ctrl Pts',(6.0061289456163,-1.24277852622533,1.52958044066593));
#34449=CARTESIAN_POINT('Ctrl Pts',(6.1379456646946,-1.93936778890619,0.424561021508401));
#34450=CARTESIAN_POINT('Ctrl Pts',(6.27066300628487,-1.79326538900601,-0.881319784202494));
#34451=CARTESIAN_POINT('Ctrl Pts',(6.40424425838086,-0.859607066663113,
-1.81773053787805));
#34452=CARTESIAN_POINT('Ctrl Pts',(6.53853932211068,0.462976199094479,-1.96763098468602));
#34453=CARTESIAN_POINT('Ctrl Pts',(6.65112996586297,1.404881072604,-1.37595823609957));
#34454=CARTESIAN_POINT('Ctrl Pts',(6.74131168525227,1.81841870776265,-0.622862303654825));
#34455=CARTESIAN_POINT('Ctrl Pts',(6.78671559508214,1.89026514761845,-0.203833176009383));
#34456=CARTESIAN_POINT('Ctrl Pts',(6.80919797775352,1.89066123052353,0.0101027673201533));
#34457=CARTESIAN_POINT('Ctrl Pts',(0.508591862447781,1.64562043801211,-0.0261324580079617));
#34458=CARTESIAN_POINT('Ctrl Pts',(0.528271024599208,1.6452737407805,0.161128837931408));
#34459=CARTESIAN_POINT('Ctrl Pts',(0.567647573513685,1.58281094560678,0.524492831752905));
#34460=CARTESIAN_POINT('Ctrl Pts',(0.645996560435206,1.22365592193525,1.1787804941138));
#34461=CARTESIAN_POINT('Ctrl Pts',(0.743073641882897,0.410281924307437,
1.68766009875447));
#34462=CARTESIAN_POINT('Ctrl Pts',(0.858352417401347,-0.724396860085975,
1.55831173688398));
#34463=CARTESIAN_POINT('Ctrl Pts',(0.972375295448021,-1.52098532662473,
0.758217612597792));
#34464=CARTESIAN_POINT('Ctrl Pts',(1.08519171777668,-1.64409811634449,-0.352032188510366));
#34465=CARTESIAN_POINT('Ctrl Pts',(1.19681996654867,-1.05450947578872,-1.28675893283186));
#34466=CARTESIAN_POINT('Ctrl Pts',(1.30730161177351,-0.0208333311052113,
-1.64663068201152));
#34467=CARTESIAN_POINT('Ctrl Pts',(1.40452364629174,0.886236470079679,-1.32621345051066));
#34468=CARTESIAN_POINT('Ctrl Pts',(1.48890750188156,1.38959463750653,-0.691912415510853));
#34469=CARTESIAN_POINT('Ctrl Pts',(1.56078188611823,1.54308896603543,-0.0198177610475133));
#34470=CARTESIAN_POINT('Ctrl Pts',(1.63221817171176,1.38983552550406,0.647948130516392));
#34471=CARTESIAN_POINT('Ctrl Pts',(1.70323404319384,0.964738946565908,1.1812205675546));
#34472=CARTESIAN_POINT('Ctrl Pts',(1.77384798276294,0.354991450441324,1.47260961294232));
#34473=CARTESIAN_POINT('Ctrl Pts',(1.86748993119896,-0.546099502039117,
1.47825694934893));
#34474=CARTESIAN_POINT('Ctrl Pts',(1.98363667823136,-1.48203264186415,0.7293081873873));
#34475=CARTESIAN_POINT('Ctrl Pts',(2.09871900316068,-1.48120258062414,-0.462340692211473));
#34476=CARTESIAN_POINT('Ctrl Pts',(2.19023826573612,-0.927379733426102,
-1.14481302651884));
#34477=CARTESIAN_POINT('Ctrl Pts',(2.2814255547235,-0.141378759287938,-1.52891931607764));
#34478=CARTESIAN_POINT('Ctrl Pts',(2.39484749559815,1.00382275253285,-1.27061478852019));
#34479=CARTESIAN_POINT('Ctrl Pts',(2.53025681997088,1.60865186335246,-0.00254459019504153));
#34480=CARTESIAN_POINT('Ctrl Pts',(2.64269039045238,1.10418776314993,1.04117197496908));
#34481=CARTESIAN_POINT('Ctrl Pts',(2.73249952801582,0.322974585676589,1.41105820876749));
#34482=CARTESIAN_POINT('Ctrl Pts',(2.7998141074244,-0.32110895921182,1.41232437949226));
#34483=CARTESIAN_POINT('Ctrl Pts',(2.86711382621074,-0.903428721470414,
1.13164638734841));
#34484=CARTESIAN_POINT('Ctrl Pts',(2.93442516377676,-1.30601623783849,0.626923391067463));
#34485=CARTESIAN_POINT('Ctrl Pts',(3.00177556402078,-1.44931171614156,-0.00280700337714968));
#34486=CARTESIAN_POINT('Ctrl Pts',(3.08042754178598,-1.28252605621248,-0.73905091180395));
#34487=CARTESIAN_POINT('Ctrl Pts',(3.17046965462109,-0.654511755766728,
-1.3704712298758));
#34488=CARTESIAN_POINT('Ctrl Pts',(3.27206448378161,0.346719679199525,-1.483704431146));
#34489=CARTESIAN_POINT('Ctrl Pts',(3.3740442463093,1.20102786916375,-0.946430056825302));
#34490=CARTESIAN_POINT('Ctrl Pts',(3.47649477143674,1.53732148053407,0.0107120740773195));
#34491=CARTESIAN_POINT('Ctrl Pts',(3.57949954098879,1.20134163447082,0.973667458417707));
#34492=CARTESIAN_POINT('Ctrl Pts',(3.68313928551533,0.333095090941954,1.52059902024328));
#34493=CARTESIAN_POINT('Ctrl Pts',(3.78749120379714,-0.693842597912142,
1.40614340263662));
#34494=CARTESIAN_POINT('Ctrl Pts',(3.89262893585172,-1.43094857905026,0.670971912346831));
#34495=CARTESIAN_POINT('Ctrl Pts',(3.99862203011025,-1.5499543985351,-0.371794281933162));
#34496=CARTESIAN_POINT('Ctrl Pts',(4.10553567293418,-0.988090997030439,
-1.26903707993744));
#34497=CARTESIAN_POINT('Ctrl Pts',(4.21343045112327,0.0197202801860453,
-1.62347464599002));
#34498=CARTESIAN_POINT('Ctrl Pts',(4.32236196180067,1.03832038776908,-1.26894288895586));
#34499=CARTESIAN_POINT('Ctrl Pts',(4.43238051112357,1.61925828890368,-0.34739423883176));
#34500=CARTESIAN_POINT('Ctrl Pts',(4.54353062752128,1.4989897755625,0.74620181404568));
#34501=CARTESIAN_POINT('Ctrl Pts',(4.65585125526312,0.71351870218781,1.53444845290457));
#34502=CARTESIAN_POINT('Ctrl Pts',(4.75676135685292,-0.279697500338493,
1.64729603227415));
#34503=CARTESIAN_POINT('Ctrl Pts',(4.84585493867587,-1.04780204615629,1.27474307821934));
#34504=CARTESIAN_POINT('Ctrl Pts',(4.94841313843452,-1.66845031883017,0.508931034591464));
#34505=CARTESIAN_POINT('Ctrl Pts',(5.07800659502253,-1.67475443904525,-0.829467776745351));
#34506=CARTESIAN_POINT('Ctrl Pts',(5.23577771702336,-0.399579932550961,
-1.85373353020478));
#34507=CARTESIAN_POINT('Ctrl Pts',(5.39581269472486,1.21472097060722,-1.48922395511139));
#34508=CARTESIAN_POINT('Ctrl Pts',(5.55809610080897,1.95203227446324,0.0217272724024816));
#34509=CARTESIAN_POINT('Ctrl Pts',(5.70888367040444,1.27533356599845,1.42745494534175));
#34510=CARTESIAN_POINT('Ctrl Pts',(5.84753617842438,-0.0234051752573978,
1.87960329280061));
#34511=CARTESIAN_POINT('Ctrl Pts',(5.9735033792588,-1.2000636353636,1.47084402209574));
#34512=CARTESIAN_POINT('Ctrl Pts',(6.10061934653175,-1.87205652425054,0.4054527917675));
#34513=CARTESIAN_POINT('Ctrl Pts',(6.22882892874595,-1.73128184695155,-0.856020464879398));
#34514=CARTESIAN_POINT('Ctrl Pts',(6.35811249074499,-0.82796691613823,-1.76256406416465));
#34515=CARTESIAN_POINT('Ctrl Pts',(6.48835538046169,0.454518312141212,-1.90827828922266));
#34516=CARTESIAN_POINT('Ctrl Pts',(6.59776527270895,1.37009311469038,-1.33377327146165));
#34517=CARTESIAN_POINT('Ctrl Pts',(6.68557306476182,1.77276616876359,-0.600525447669764));
#34518=CARTESIAN_POINT('Ctrl Pts',(6.72979494253028,1.84279755540219,-0.192431284750887));
#34519=CARTESIAN_POINT('Ctrl Pts',(6.75172308477496,1.84318387398818,0.016230664703078));
#34520=CARTESIAN_POINT('',(0.508591862447781,1.64562043801211,-0.0261324580079617));
#34521=CARTESIAN_POINT('Origin',(0.26,1.65,1.37288700589905E-18));
#34522=CARTESIAN_POINT('',(6.75172308477496,1.84318387398818,0.016230664703078));
#34523=CARTESIAN_POINT('Ctrl Pts',(0.508591862447781,1.64562043801211,-0.0261324580079617));
#34524=CARTESIAN_POINT('Ctrl Pts',(0.528271024599208,1.6452737407805,0.161128837931408));
#34525=CARTESIAN_POINT('Ctrl Pts',(0.567647573513685,1.58281094560678,0.524492831752905));
#34526=CARTESIAN_POINT('Ctrl Pts',(0.645996560435206,1.22365592193525,1.1787804941138));
#34527=CARTESIAN_POINT('Ctrl Pts',(0.743073641882897,0.410281924307437,
1.68766009875447));
#34528=CARTESIAN_POINT('Ctrl Pts',(0.858352417401347,-0.724396860085975,
1.55831173688398));
#34529=CARTESIAN_POINT('Ctrl Pts',(0.972375295448021,-1.52098532662473,
0.758217612597792));
#34530=CARTESIAN_POINT('Ctrl Pts',(1.08519171777668,-1.64409811634449,-0.352032188510366));
#34531=CARTESIAN_POINT('Ctrl Pts',(1.19681996654867,-1.05450947578872,-1.28675893283186));
#34532=CARTESIAN_POINT('Ctrl Pts',(1.30730161177351,-0.0208333311052113,
-1.64663068201152));
#34533=CARTESIAN_POINT('Ctrl Pts',(1.40452364629174,0.886236470079679,-1.32621345051066));
#34534=CARTESIAN_POINT('Ctrl Pts',(1.48890750188156,1.38959463750653,-0.691912415510853));
#34535=CARTESIAN_POINT('Ctrl Pts',(1.56078188611823,1.54308896603543,-0.0198177610475133));
#34536=CARTESIAN_POINT('Ctrl Pts',(1.63221817171176,1.38983552550406,0.647948130516392));
#34537=CARTESIAN_POINT('Ctrl Pts',(1.70323404319384,0.964738946565908,1.1812205675546));
#34538=CARTESIAN_POINT('Ctrl Pts',(1.77384798276294,0.354991450441324,1.47260961294232));
#34539=CARTESIAN_POINT('Ctrl Pts',(1.86748993119896,-0.546099502039117,
1.47825694934893));
#34540=CARTESIAN_POINT('Ctrl Pts',(1.98363667823136,-1.48203264186415,0.7293081873873));
#34541=CARTESIAN_POINT('Ctrl Pts',(2.09871900316068,-1.48120258062414,-0.462340692211473));
#34542=CARTESIAN_POINT('Ctrl Pts',(2.19023826573612,-0.927379733426102,
-1.14481302651884));
#34543=CARTESIAN_POINT('Ctrl Pts',(2.2814255547235,-0.141378759287938,-1.52891931607764));
#34544=CARTESIAN_POINT('Ctrl Pts',(2.39484749559815,1.00382275253285,-1.27061478852019));
#34545=CARTESIAN_POINT('Ctrl Pts',(2.53025681997088,1.60865186335246,-0.00254459019504153));
#34546=CARTESIAN_POINT('Ctrl Pts',(2.64269039045238,1.10418776314993,1.04117197496908));
#34547=CARTESIAN_POINT('Ctrl Pts',(2.73249952801582,0.322974585676589,1.41105820876749));
#34548=CARTESIAN_POINT('Ctrl Pts',(2.7998141074244,-0.32110895921182,1.41232437949226));
#34549=CARTESIAN_POINT('Ctrl Pts',(2.86711382621074,-0.903428721470414,
1.13164638734841));
#34550=CARTESIAN_POINT('Ctrl Pts',(2.93442516377676,-1.30601623783849,0.626923391067463));
#34551=CARTESIAN_POINT('Ctrl Pts',(3.00177556402078,-1.44931171614156,-0.00280700337714968));
#34552=CARTESIAN_POINT('Ctrl Pts',(3.08042754178598,-1.28252605621248,-0.73905091180395));
#34553=CARTESIAN_POINT('Ctrl Pts',(3.17046965462109,-0.654511755766728,
-1.3704712298758));
#34554=CARTESIAN_POINT('Ctrl Pts',(3.27206448378161,0.346719679199525,-1.483704431146));
#34555=CARTESIAN_POINT('Ctrl Pts',(3.3740442463093,1.20102786916375,-0.946430056825302));
#34556=CARTESIAN_POINT('Ctrl Pts',(3.47649477143674,1.53732148053407,0.0107120740773195));
#34557=CARTESIAN_POINT('Ctrl Pts',(3.57949954098879,1.20134163447082,0.973667458417707));
#34558=CARTESIAN_POINT('Ctrl Pts',(3.68313928551533,0.333095090941954,1.52059902024328));
#34559=CARTESIAN_POINT('Ctrl Pts',(3.78749120379714,-0.693842597912142,
1.40614340263662));
#34560=CARTESIAN_POINT('Ctrl Pts',(3.89262893585172,-1.43094857905026,0.670971912346831));
#34561=CARTESIAN_POINT('Ctrl Pts',(3.99862203011025,-1.5499543985351,-0.371794281933162));
#34562=CARTESIAN_POINT('Ctrl Pts',(4.10553567293418,-0.988090997030439,
-1.26903707993744));
#34563=CARTESIAN_POINT('Ctrl Pts',(4.21343045112327,0.0197202801860453,
-1.62347464599002));
#34564=CARTESIAN_POINT('Ctrl Pts',(4.32236196180067,1.03832038776908,-1.26894288895586));
#34565=CARTESIAN_POINT('Ctrl Pts',(4.43238051112357,1.61925828890368,-0.34739423883176));
#34566=CARTESIAN_POINT('Ctrl Pts',(4.54353062752128,1.4989897755625,0.74620181404568));
#34567=CARTESIAN_POINT('Ctrl Pts',(4.65585125526312,0.71351870218781,1.53444845290457));
#34568=CARTESIAN_POINT('Ctrl Pts',(4.75676135685292,-0.279697500338493,
1.64729603227415));
#34569=CARTESIAN_POINT('Ctrl Pts',(4.84585493867587,-1.04780204615629,1.27474307821934));
#34570=CARTESIAN_POINT('Ctrl Pts',(4.94841313843452,-1.66845031883017,0.508931034591464));
#34571=CARTESIAN_POINT('Ctrl Pts',(5.07800659502253,-1.67475443904525,-0.829467776745351));
#34572=CARTESIAN_POINT('Ctrl Pts',(5.23577771702336,-0.399579932550961,
-1.85373353020478));
#34573=CARTESIAN_POINT('Ctrl Pts',(5.39581269472486,1.21472097060722,-1.48922395511139));
#34574=CARTESIAN_POINT('Ctrl Pts',(5.55809610080897,1.95203227446324,0.0217272724024816));
#34575=CARTESIAN_POINT('Ctrl Pts',(5.70888367040444,1.27533356599845,1.42745494534175));
#34576=CARTESIAN_POINT('Ctrl Pts',(5.84753617842438,-0.0234051752573978,
1.87960329280061));
#34577=CARTESIAN_POINT('Ctrl Pts',(5.9735033792588,-1.2000636353636,1.47084402209574));
#34578=CARTESIAN_POINT('Ctrl Pts',(6.10061934653175,-1.87205652425054,0.4054527917675));
#34579=CARTESIAN_POINT('Ctrl Pts',(6.22882892874595,-1.73128184695155,-0.856020464879398));
#34580=CARTESIAN_POINT('Ctrl Pts',(6.35811249074499,-0.82796691613823,-1.76256406416465));
#34581=CARTESIAN_POINT('Ctrl Pts',(6.48835538046169,0.454518312141212,-1.90827828922266));
#34582=CARTESIAN_POINT('Ctrl Pts',(6.59776527270895,1.37009311469038,-1.33377327146165));
#34583=CARTESIAN_POINT('Ctrl Pts',(6.68557306476182,1.77276616876359,-0.600525447669764));
#34584=CARTESIAN_POINT('Ctrl Pts',(6.72979494253028,1.84279755540219,-0.192431284750887));
#34585=CARTESIAN_POINT('Ctrl Pts',(6.75172308477496,1.84318387398818,0.016230664703078));
#34586=CARTESIAN_POINT('Origin',(6.90957287525381,1.65,-2.42861286636753E-15));
#34587=CARTESIAN_POINT('Origin',(6.90957287525381,1.65,-2.42861286636753E-15));
#34588=CARTESIAN_POINT('Origin',(0.26,1.65,1.37288700589905E-18));
#38511=UNCERTAINTY_MEASURE_WITH_UNIT(LENGTH_MEASURE(0.01),#38529,
'DISTANCE_ACCURACY_VALUE',
'Maximum model space distance between geometric entities at asserted c
onnectivities');
#38514=UNCERTAINTY_MEASURE_WITH_UNIT(LENGTH_MEASURE(0.01),#38529,
'DISTANCE_ACCURACY_VALUE',
'Maximum model space distance between geometric entities at asserted c
onnectivities');
#38525=(
GEOMETRIC_REPRESENTATION_CONTEXT(3)
GLOBAL_UNCERTAINTY_ASSIGNED_CONTEXT((#38511))
GLOBAL_UNIT_ASSIGNED_CONTEXT((#38529,#38531,#38532))
REPRESENTATION_CONTEXT('','3D')
);
#38528=(
GEOMETRIC_REPRESENTATION_CONTEXT(3)
GLOBAL_UNCERTAINTY_ASSIGNED_CONTEXT((#38514))
GLOBAL_UNIT_ASSIGNED_CONTEXT((#38529,#38531,#38532))
REPRESENTATION_CONTEXT('','3D')
);
#38529=(
LENGTH_UNIT()
NAMED_UNIT(*)
SI_UNIT(.MILLI.,.METRE.)
);
#38531=(
NAMED_UNIT(*)
PLANE_ANGLE_UNIT()
SI_UNIT($,.RADIAN.)
);
#38532=(
NAMED_UNIT(*)
SI_UNIT($,.STERADIAN.)
SOLID_ANGLE_UNIT()
);
#38543=SHAPE_DEFINITION_REPRESENTATION(#38556,#38585);
#38556=PRODUCT_DEFINITION_SHAPE('',$,#38599);
#38585=SHAPE_REPRESENTATION('',(#18769),#38525);
#38588=PRODUCT_DEFINITION_CONTEXT('part definition',#38629,'design');
#38599=PRODUCT_DEFINITION('2026-10-20-13-39-10-551',
'10_Detent_Spring_D3.8',#38612,#38588);
#38612=PRODUCT_DEFINITION_FORMATION('',$,#38641);
#38629=APPLICATION_CONTEXT(
'Core Data for Automotive Mechanical Design Process');
#38630=PRODUCT_CONTEXT('part definition',#38629,'mechanical');
#38641=PRODUCT('2026-10-20-13-39-10-551','10_Detent_Spring_D3.8',$,(#38630));
#38700=COLOUR_RGB('Grey',0.48,0.52,0.57);
#38701=FILL_AREA_STYLE_COLOUR('',#38700);
#38702=FILL_AREA_STYLE('',(#38701));
#38703=SURFACE_STYLE_FILL_AREA(#38702);
#38704=SURFACE_SIDE_STYLE('',(#38703));
#38705=SURFACE_STYLE_USAGE(.BOTH.,#38704);
#38706=PRESENTATION_STYLE_ASSIGNMENT((#38705));
ENDSEC;
END-ISO-10303-21;
